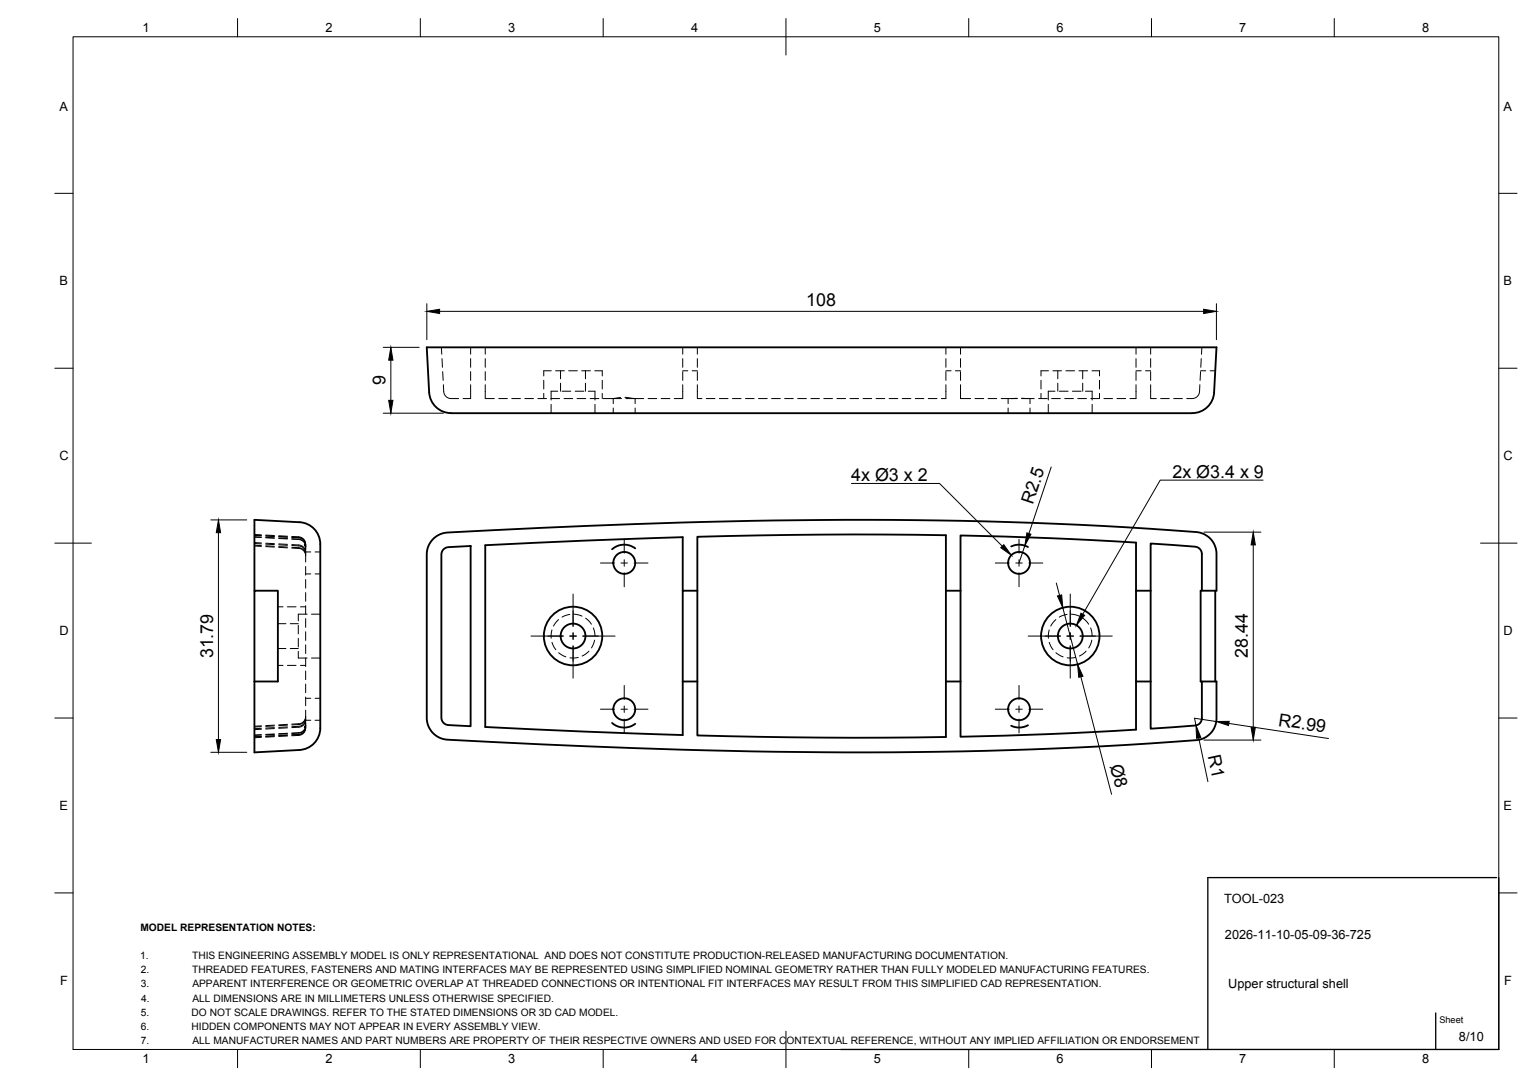
ISO-10303-21;
HEADER;
/* Generated by software containing ST-Developer
 * from STEP Tools, Inc. (www.steptools.com) 
 */

FILE_DESCRIPTION(
/* description */ (''),
/* implementation_level */ '2;1');

FILE_NAME(
/* name */ 'Upper structural shell.step',
/* time_stamp */ '2026-11-10T05:40:20-08:00',
/* author */ (''),
/* organization */ (''),
/* preprocessor_version */ 'ST-DEVELOPER v20.2',
/* originating_system */ 'Autodesk Translation Framework v15.17.0.0',
/* authorisation */ '');

FILE_SCHEMA (('AUTOMOTIVE_DESIGN { 1 0 10303 214 3 1 1 }'));
ENDSEC;

DATA;
#10=MECHANICAL_DESIGN_GEOMETRIC_PRESENTATION_REPRESENTATION('',(#575),#18580);
#76=SPHERICAL_SURFACE('',#6795,0.1);
#77=SPHERICAL_SURFACE('',#6798,0.0999999999999998);
#78=SPHERICAL_SURFACE('',#6802,0.0999999999999993);
#79=SPHERICAL_SURFACE('',#6806,0.1);
#80=SPHERICAL_SURFACE('',#6811,0.3);
#81=SPHERICAL_SURFACE('',#6815,0.3);
#82=SPHERICAL_SURFACE('',#6819,0.299999999999999);
#83=SPHERICAL_SURFACE('',#6824,0.3);
#92=B_SPLINE_SURFACE_WITH_KNOTS('',3,3,((#8816,#8817,#8818,#8819),(#8820,
#8821,#8822,#8823),(#8824,#8825,#8826,#8827),(#8828,#8829,#8830,#8831),
(#8832,#8833,#8834,#8835)),.UNSPECIFIED.,.F.,.F.,.F.,(4,1,4),(4,4),(0.,
0.571428571428571,1.),(1.0454440030657,3.44967454744645),.UNSPECIFIED.);
#93=B_SPLINE_SURFACE_WITH_KNOTS('',3,3,((#8908,#8909,#8910,#8911),(#8912,
#8913,#8914,#8915),(#8916,#8917,#8918,#8919),(#8920,#8921,#8922,#8923),
(#8924,#8925,#8926,#8927)),.UNSPECIFIED.,.F.,.F.,.F.,(4,1,4),(4,4),(0.,
0.571428571428571,1.),(7.24519303641511,9.95046872158573),.UNSPECIFIED.);
#94=B_SPLINE_SURFACE_WITH_KNOTS('',3,3,((#9789,#9790,#9791,#9792),(#9793,
#9794,#9795,#9796),(#9797,#9798,#9799,#9800),(#9801,#9802,#9803,#9804)),
 .UNSPECIFIED.,.F.,.F.,.F.,(4,4),(4,4),(0.0705535719740953,0.323522444336189),
(0.0117434863834119,0.684857763552191),.UNSPECIFIED.);
#95=B_SPLINE_SURFACE_WITH_KNOTS('',3,3,((#9809,#9810,#9811,#9812),(#9813,
#9814,#9815,#9816),(#9817,#9818,#9819,#9820),(#9821,#9822,#9823,#9824)),
 .UNSPECIFIED.,.F.,.F.,.F.,(4,4),(4,4),(0.0262419052680539,0.0545428296147404),
(0.0121538053864343,0.684980602226481),.UNSPECIFIED.);
#96=B_SPLINE_SURFACE_WITH_KNOTS('',3,3,((#9834,#9835,#9836,#9837),(#9838,
#9839,#9840,#9841),(#9842,#9843,#9844,#9845),(#9846,#9847,#9848,#9849),
(#9850,#9851,#9852,#9853)),.UNSPECIFIED.,.F.,.F.,.F.,(4,1,4),(4,4),(0.,
0.571428571428571,1.),(0.752061768057538,3.45733745322815),
 .UNSPECIFIED.);
#97=B_SPLINE_SURFACE_WITH_KNOTS('',3,3,((#9854,#9855,#9856,#9857),(#9858,
#9859,#9860,#9861),(#9862,#9863,#9864,#9865),(#9866,#9867,#9868,#9869),
(#9870,#9871,#9872,#9873)),.UNSPECIFIED.,.F.,.F.,.F.,(4,1,4),(4,4),(0.,
0.571428571428571,1.),(0.283259008618247,0.557056952888827),
 .UNSPECIFIED.);
#98=B_SPLINE_SURFACE_WITH_KNOTS('',3,3,((#9887,#9888,#9889,#9890),(#9891,
#9892,#9893,#9894),(#9895,#9896,#9897,#9898),(#9899,#9900,#9901,#9902)),
 .UNSPECIFIED.,.F.,.F.,.F.,(4,4),(4,4),(0.67647755566375,0.929446428026011),
(0.0117434863436937,0.684857763580381),.UNSPECIFIED.);
#99=B_SPLINE_SURFACE_WITH_KNOTS('',3,3,((#9903,#9904,#9905,#9906),(#9907,
#9908,#9909,#9910),(#9911,#9912,#9913,#9914),(#9915,#9916,#9917,#9918)),
 .UNSPECIFIED.,.F.,.F.,.F.,(4,4),(4,4),(0.945457170385156,0.973758094731946),
(0.0121538053598088,0.684980602226481),.UNSPECIFIED.);
#100=B_SPLINE_SURFACE_WITH_KNOTS('',3,3,((#10002,#10003,#10004,#10005),
(#10006,#10007,#10008,#10009),(#10010,#10011,#10012,#10013),(#10014,#10015,
#10016,#10017)),.UNSPECIFIED.,.F.,.F.,.F.,(4,4),(4,4),(0.341142793678372,
0.658675488550287),(0.0116221239297273,0.684255166525269),.UNSPECIFIED.);
#101=B_SPLINE_SURFACE_WITH_KNOTS('',3,3,((#10022,#10023,#10024,#10025),
(#10026,#10027,#10028,#10029),(#10030,#10031,#10032,#10033),(#10034,#10035,
#10036,#10037),(#10038,#10039,#10040,#10041)),.UNSPECIFIED.,.F.,.F.,.F.,
(4,1,4),(4,4),(0.,0.571428571428571,1.),(3.65450559744172,7.0548588409572),
 .UNSPECIFIED.);
#102=B_SPLINE_SURFACE_WITH_KNOTS('',3,3,((#10051,#10052,#10053,#10054),
(#10055,#10056,#10057,#10058),(#10059,#10060,#10061,#10062),(#10063,#10064,
#10065,#10066),(#10067,#10068,#10069,#10070)),.UNSPECIFIED.,.F.,.F.,.F.,
(4,1,4),(4,4),(0.,0.571428571428571,1.),(3.64767164868607,7.04802489220155),
 .UNSPECIFIED.);
#103=B_SPLINE_SURFACE_WITH_KNOTS('',3,3,((#10075,#10076,#10077,#10078),
(#10079,#10080,#10081,#10082),(#10083,#10084,#10085,#10086),(#10087,#10088,
#10089,#10090)),.UNSPECIFIED.,.F.,.F.,.F.,(4,4),(4,4),(0.341324511449716,
0.658857206321627),(0.0116221214776208,0.684255166525269),.UNSPECIFIED.);
#104=B_SPLINE_SURFACE_WITH_KNOTS('',3,3,((#10135,#10136,#10137,#10138),
(#10139,#10140,#10141,#10142),(#10143,#10144,#10145,#10146),(#10147,#10148,
#10149,#10150)),.UNSPECIFIED.,.F.,.F.,.F.,(4,4),(4,4),(0.676316266718331,
0.901708040522105),(0.0117102006467275,0.68495201331719),.UNSPECIFIED.);
#105=B_SPLINE_SURFACE_WITH_KNOTS('',3,3,((#10155,#10156,#10157,#10158),
(#10159,#10160,#10161,#10162),(#10163,#10164,#10165,#10166),(#10167,#10168,
#10169,#10170),(#10171,#10172,#10173,#10174)),.UNSPECIFIED.,.F.,.F.,.F.,
(4,1,4),(4,4),(0.,0.571428571428571,1.),(7.25285594219682,9.65708648657758),
 .UNSPECIFIED.);
#106=B_SPLINE_SURFACE_WITH_KNOTS('',3,3,((#10184,#10185,#10186,#10187),
(#10188,#10189,#10190,#10191),(#10192,#10193,#10194,#10195),(#10196,#10197,
#10198,#10199)),.UNSPECIFIED.,.F.,.F.,.F.,(4,4),(4,4),(0.0982919594778951,
0.323683733281714),(0.0117102006467272,0.68495201331719),.UNSPECIFIED.);
#107=B_SPLINE_SURFACE_WITH_KNOTS('',3,3,((#10274,#10275,#10276,#10277),
(#10278,#10279,#10280,#10281),(#10282,#10283,#10284,#10285),(#10286,#10287,
#10288,#10289)),.UNSPECIFIED.,.F.,.F.,.F.,(4,4),(4,4),(0.917922863855343,
0.974411608827007),(0.0122403473423911,0.685344304754238),.UNSPECIFIED.);
#108=B_SPLINE_SURFACE_WITH_KNOTS('',3,3,((#10299,#10300,#10301,#10302),
(#10303,#10304,#10305,#10306),(#10307,#10308,#10309,#10310),(#10311,#10312,
#10313,#10314),(#10315,#10316,#10317,#10318)),.UNSPECIFIED.,.F.,.F.,.F.,
(4,1,4),(4,4),(0.,0.571428571428571,1.),(9.85085636625011,10.4271318523291),
 .UNSPECIFIED.);
#109=B_SPLINE_SURFACE_WITH_KNOTS('',3,3,((#10332,#10333,#10334,#10335),
(#10336,#10337,#10338,#10339),(#10340,#10341,#10342,#10343),(#10344,#10345,
#10346,#10347)),.UNSPECIFIED.,.F.,.F.,.F.,(4,4),(4,4),(0.025588391172993,
0.0820771361446569),(0.0122403473423911,0.685344304754238),
 .UNSPECIFIED.);
#110=B_SPLINE_SURFACE_WITH_KNOTS('',3,3,((#10357,#10358,#10359,#10360),
(#10361,#10362,#10363,#10364),(#10365,#10366,#10367,#10368),(#10369,#10370,
#10371,#10372),(#10373,#10374,#10375,#10376)),.UNSPECIFIED.,.F.,.F.,.F.,
(4,1,4),(4,4),(0.,0.571428571428571,1.),(0.27539863731415,0.851674123393175),
 .UNSPECIFIED.);
#111=B_SPLINE_SURFACE_WITH_KNOTS('',3,3,((#10390,#10391,#10392,#10393),
(#10394,#10395,#10396,#10397),(#10398,#10399,#10400,#10401),(#10402,#10403,
#10404,#10405),(#10406,#10407,#10408,#10409)),.UNSPECIFIED.,.F.,.F.,.F.,
(4,1,4),(4,4),(0.,0.571428571428571,1.),(0.00944995813270487,0.618489359031386),
 .UNSPECIFIED.);
#112=B_SPLINE_SURFACE_WITH_KNOTS('',3,3,((#10416,#10417,#10418,#10419),
(#10420,#10421,#10422,#10423),(#10424,#10425,#10426,#10427),(#10428,#10429,
#10430,#10431),(#10432,#10433,#10434,#10435)),.UNSPECIFIED.,.F.,.F.,.F.,
(4,1,4),(4,4),(0.,0.571428571428571,1.),(0.00908570715245136,0.618164468641375),
 .UNSPECIFIED.);
#113=B_SPLINE_SURFACE_WITH_KNOTS('',3,3,((#10440,#10441,#10442,#10443),
(#10444,#10445,#10446,#10447),(#10448,#10449,#10450,#10451),(#10452,#10453,
#10454,#10455),(#10456,#10457,#10458,#10459)),.UNSPECIFIED.,.F.,.F.,.F.,
(4,1,4),(4,4),(0.,0.571428571428571,1.),(0.0091183540525243,0.618164468641375),
 .UNSPECIFIED.);
#114=B_SPLINE_SURFACE_WITH_KNOTS('',3,3,((#10464,#10465,#10466,#10467),
(#10468,#10469,#10470,#10471),(#10472,#10473,#10474,#10475),(#10476,#10477,
#10478,#10479),(#10480,#10481,#10482,#10483)),.UNSPECIFIED.,.F.,.F.,.F.,
(4,1,4),(4,4),(0.,0.571428571428571,1.),(10.1454735367545,10.419271481025),
 .UNSPECIFIED.);
#115=B_SPLINE_SURFACE_WITH_KNOTS('',3,3,((#10484,#10485,#10486,#10487),
(#10488,#10489,#10490,#10491),(#10492,#10493,#10494,#10495),(#10496,#10497,
#10498,#10499),(#10500,#10501,#10502,#10503)),.UNSPECIFIED.,.F.,.F.,.F.,
(4,1,4),(4,4),(0.,0.571428571428571,1.),(0.0094045468285345,0.618489359031386),
 .UNSPECIFIED.);
#116=B_SPLINE_SURFACE_WITH_KNOTS('',3,3,((#10529,#10530,#10531,#10532),
(#10533,#10534,#10535,#10536),(#10537,#10538,#10539,#10540),(#10541,#10542,
#10543,#10544),(#10545,#10546,#10547,#10548)),.UNSPECIFIED.,.F.,.F.,.F.,
(4,1,4),(4,4),(0.,0.571428571428571,1.),(-0.00535061636073277,0.618489359031386),
 .UNSPECIFIED.);
#117=B_SPLINE_SURFACE_WITH_KNOTS('',3,3,((#10567,#10568,#10569,#10570,#10571),
(#10572,#10573,#10574,#10575,#10576),(#10577,#10578,#10579,#10580,#10581),
(#10582,#10583,#10584,#10585,#10586),(#10587,#10588,#10589,#10590,#10591)),
 .UNSPECIFIED.,.F.,.F.,.F.,(4,1,4),(4,1,4),(0.,0.571428571428571,1.),(0.283259008618247,
4.63063308449434,10.4271318523291),.UNSPECIFIED.);
#118=B_SPLINE_SURFACE_WITH_KNOTS('',3,3,((#10602,#10603,#10604,#10605),
(#10606,#10607,#10608,#10609),(#10610,#10611,#10612,#10613),(#10614,#10615,
#10616,#10617),(#10618,#10619,#10620,#10621)),.UNSPECIFIED.,.F.,.F.,.F.,
(4,1,4),(4,4),(0.,0.571428571428571,1.),(-0.00578978989683084,0.618164468641375),
 .UNSPECIFIED.);
#119=B_SPLINE_SURFACE_WITH_KNOTS('',3,3,((#10630,#10631,#10632,#10633),
(#10634,#10635,#10636,#10637),(#10638,#10639,#10640,#10641),(#10642,#10643,
#10644,#10645),(#10646,#10647,#10648,#10649)),.UNSPECIFIED.,.F.,.F.,.F.,
(4,1,4),(4,4),(0.,0.571428571428571,1.),(-0.00569189159989896,0.618164468641375),
 .UNSPECIFIED.);
#120=B_SPLINE_SURFACE_WITH_KNOTS('',3,3,((#10658,#10659,#10660,#10661,#10662),
(#10663,#10664,#10665,#10666,#10667),(#10668,#10669,#10670,#10671,#10672),
(#10673,#10674,#10675,#10676,#10677),(#10678,#10679,#10680,#10681,#10682)),
 .UNSPECIFIED.,.F.,.F.,.F.,(4,1,4),(4,1,4),(0.,0.571428571428571,1.),(0.27539863731415,
4.62277271319024,10.419271481025),.UNSPECIFIED.);
#121=B_SPLINE_SURFACE_WITH_KNOTS('',3,3,((#10693,#10694,#10695,#10696),
(#10697,#10698,#10699,#10700),(#10701,#10702,#10703,#10704),(#10705,#10706,
#10707,#10708),(#10709,#10710,#10711,#10712)),.UNSPECIFIED.,.F.,.F.,.F.,
(4,1,4),(4,4),(0.,0.571428571428571,1.),(-0.0054868135546625,0.618489359031386),
 .UNSPECIFIED.);
#122=B_SPLINE_SURFACE_WITH_KNOTS('',3,3,((#10721,#10722,#10723,#10724),
(#10725,#10726,#10727,#10728),(#10729,#10730,#10731,#10732),(#10733,#10734,
#10735,#10736)),.UNSPECIFIED.,.F.,.F.,.F.,(4,4),(4,4),(0.026239262514127,
0.974414173651419),(0.,0.685344304754238),.UNSPECIFIED.);
#123=B_SPLINE_SURFACE_WITH_KNOTS('',3,3,((#10739,#10740,#10741,#10742),
(#10743,#10744,#10745,#10746),(#10747,#10748,#10749,#10750),(#10751,#10752,
#10753,#10754)),.UNSPECIFIED.,.F.,.F.,.F.,(4,4),(4,4),(0.0255858263485814,
0.973760737485873),(0.,0.685344304754238),.UNSPECIFIED.);
#172=B_SPLINE_CURVE_WITH_KNOTS('',3,(#8715,#8716,#8717,#8718,#8719,#8720,
#8721,#8722,#8723,#8724,#8725,#8726,#8727,#8728,#8729,#8730,#8731,#8732,
#8733,#8734,#8735,#8736,#8737,#8738),.UNSPECIFIED.,.F.,.F.,(4,2,2,2,2,2,
2,2,2,2,2,4),(-0.337265338267783,-0.250544943628509,-0.208272806508042,
-0.186542211788094,-0.176382978682897,-0.170925844043069,-0.16639450677335,
-0.161077381235501,-0.15182241135393,-0.115009181549223,-0.030206004227969,
0.),.UNSPECIFIED.);
#173=B_SPLINE_CURVE_WITH_KNOTS('',3,(#8743,#8744,#8745,#8746,#8747,#8748,
#8749,#8750,#8751,#8752,#8753,#8754,#8755,#8756,#8757,#8758,#8759,#8760,
#8761,#8762),.UNSPECIFIED.,.F.,.F.,(4,2,2,2,2,2,2,2,2,4),(-0.240982594686416,
-0.16829976149504,-0.141836598208813,-0.129116059226128,-0.121962912034391,
-0.115857591426886,-0.108506552485159,-0.0948769875819265,-0.0364654790774683,
0.),.UNSPECIFIED.);
#174=B_SPLINE_CURVE_WITH_KNOTS('',3,(#8767,#8768,#8769,#8770,#8771,#8772,
#8773,#8774,#8775,#8776,#8777,#8778,#8779,#8780,#8781,#8782,#8783,#8784,
#8785,#8786),.UNSPECIFIED.,.F.,.F.,(4,2,2,2,2,2,2,2,2,4),(-0.240981214998207,
-0.168303541671295,-0.141841407502325,-0.129121097580905,-0.121968013294536,
-0.115862708924237,-0.108511643765797,-0.0948818976588229,-0.0364681276985956,
0.),.UNSPECIFIED.);
#175=B_SPLINE_CURVE_WITH_KNOTS('',3,(#8791,#8792,#8793,#8794,#8795,#8796,
#8797,#8798,#8799,#8800,#8801,#8802,#8803,#8804,#8805,#8806,#8807,#8808,
#8809,#8810,#8811,#8812,#8813,#8814),.UNSPECIFIED.,.F.,.F.,(4,2,2,2,2,2,
2,2,2,2,2,4),(-0.337269388373684,-0.250545316912909,-0.208282401844766,
-0.186554569827561,-0.176396213396297,-0.17093921790305,-0.16640782243471,
-0.161090427650893,-0.151834477986603,-0.115010808423941,-0.0302102096065556,
0.),.UNSPECIFIED.);
#176=B_SPLINE_CURVE_WITH_KNOTS('',3,(#8837,#8838,#8839,#8840),
 .UNSPECIFIED.,.F.,.F.,(4,4),(1.0454440030657,2.52465537163019),
 .UNSPECIFIED.);
#177=B_SPLINE_CURVE_WITH_KNOTS('',3,(#8842,#8843,#8844,#8845,#8846,#8847,
#8848,#8849,#8850,#8851,#8852,#8853,#8854,#8855,#8856,#8857,#8858,#8859,
#8860,#8861,#8862,#8863,#8864,#8865,#8866,#8867,#8868,#8869),
 .UNSPECIFIED.,.F.,.F.,(4,3,3,3,3,3,3,3,3,4),(-0.152193408756968,-0.128427023368412,
-0.115107736263918,-0.0911810900745799,-0.0780377802127556,-0.0652031397886901,
-0.0414031558437525,-0.0389949527774582,-0.0152076153333754,0.),
 .UNSPECIFIED.);
#178=B_SPLINE_CURVE_WITH_KNOTS('',3,(#8871,#8872,#8873,#8874),
 .UNSPECIFIED.,.F.,.F.,(4,4),(-3.44967454744645,-1.05170160817356),
 .UNSPECIFIED.);
#179=B_SPLINE_CURVE_WITH_KNOTS('',3,(#8876,#8877,#8878,#8879,#8880,#8881,
#8882,#8883,#8884,#8885,#8886,#8887,#8888,#8889,#8890,#8891,#8892,#8893,
#8894,#8895,#8896,#8897,#8898,#8899,#8900,#8901,#8902,#8903),
 .UNSPECIFIED.,.F.,.F.,(4,3,3,3,3,3,3,3,3,4),(-0.152278960443096,-0.128503570101575,
-0.115218572146868,-0.09145408274965,-0.0870214650669139,-0.0781562978024333,
-0.0542566895399357,-0.03908030849237,-0.0153296112319379,0.),
 .UNSPECIFIED.);
#180=B_SPLINE_CURVE_WITH_KNOTS('',3,(#8904,#8905,#8906,#8907),
 .UNSPECIFIED.,.F.,.F.,(4,4),(2.75501813708031,3.4476340663212),
 .UNSPECIFIED.);
#181=B_SPLINE_CURVE_WITH_KNOTS('',3,(#8929,#8930,#8931,#8932),
 .UNSPECIFIED.,.F.,.F.,(4,4),(7.24810383506675,7.89761558728778),
 .UNSPECIFIED.);
#182=B_SPLINE_CURVE_WITH_KNOTS('',3,(#8934,#8935,#8936,#8937,#8938,#8939,
#8940,#8941,#8942,#8943,#8944,#8945,#8946,#8947,#8948,#8949,#8950,#8951,
#8952,#8953,#8954,#8955,#8956,#8957,#8958,#8959,#8960,#8961),
 .UNSPECIFIED.,.F.,.F.,(4,3,3,3,3,3,3,3,3,4),(-0.152278869104567,-0.128548794904564,
-0.115192257893812,-0.0912773536606376,-0.0781090575823055,-0.0652724057916263,
-0.0414819581560496,-0.0390493575290778,-0.015259721743698,0.),
 .UNSPECIFIED.);
#183=B_SPLINE_CURVE_WITH_KNOTS('',3,(#8963,#8964,#8965,#8966),
 .UNSPECIFIED.,.F.,.F.,(4,4),(-9.94532343034734,-7.24519303641511),
 .UNSPECIFIED.);
#184=B_SPLINE_CURVE_WITH_KNOTS('',3,(#8968,#8969,#8970,#8971,#8972,#8973,
#8974,#8975,#8976,#8977,#8978,#8979,#8980,#8981,#8982,#8983,#8984,#8985,
#8986,#8987,#8988,#8989,#8990,#8991,#8992,#8993,#8994,#8995),
 .UNSPECIFIED.,.F.,.F.,(4,3,3,3,3,3,3,3,3,4),(-0.152181623618259,-0.128410404494075,
-0.115248188224843,-0.0914746846046984,-0.0869904866333268,-0.0783028696190655,
-0.0543945376065823,-0.0391651209697638,-0.0153884182770307,0.),
 .UNSPECIFIED.);
#185=B_SPLINE_CURVE_WITH_KNOTS('',3,(#8996,#8997,#8998,#8999),
 .UNSPECIFIED.,.F.,.F.,(4,4),(8.21380824320284,9.95046871680089),
 .UNSPECIFIED.);
#186=B_SPLINE_CURVE_WITH_KNOTS('',3,(#9002,#9003,#9004,#9005),
 .UNSPECIFIED.,.F.,.F.,(4,4),(2.80491490332713,3.45442665446657),
 .UNSPECIFIED.);
#187=B_SPLINE_CURVE_WITH_KNOTS('',3,(#9009,#9010,#9011,#9012),
 .UNSPECIFIED.,.F.,.F.,(4,4),(0.752061768057538,2.48872224644044),
 .UNSPECIFIED.);
#188=B_SPLINE_CURVE_WITH_KNOTS('',3,(#9160,#9161,#9162,#9163,#9164,#9165),
 .UNSPECIFIED.,.F.,.F.,(4,2,4),(-0.606700505977711,-0.303383635264422,-0.000339350725729326),
 .UNSPECIFIED.);
#189=B_SPLINE_CURVE_WITH_KNOTS('',3,(#9166,#9167,#9168,#9169,#9170,#9171,
#9172,#9173,#9174,#9175,#9176,#9177,#9178,#9179,#9180,#9181,#9182,#9183,
#9184,#9185,#9186,#9187,#9188,#9189,#9190,#9191,#9192,#9193),
 .UNSPECIFIED.,.F.,.F.,(4,3,3,3,3,3,3,3,3,4),(-0.152173579228948,-0.128423230539522,
-0.115115104157663,-0.0911927259648815,-0.0780672068328041,-0.0652082609452843,
-0.0414117413801899,-0.0390174000215468,-0.0152300060615686,0.),
 .UNSPECIFIED.);
#190=B_SPLINE_CURVE_WITH_KNOTS('',3,(#9194,#9195,#9196,#9197,#9198,#9199),
 .UNSPECIFIED.,.F.,.F.,(4,2,4),(-0.606471894652381,-0.303383500305553,-0.00011071898471493),
 .UNSPECIFIED.);
#191=B_SPLINE_CURVE_WITH_KNOTS('',3,(#9203,#9204,#9205,#9206,#9207,#9208),
 .UNSPECIFIED.,.F.,.F.,(4,2,4),(-0.606240625011114,-0.303433113375332,-0.00010938105916114),
 .UNSPECIFIED.);
#192=B_SPLINE_CURVE_WITH_KNOTS('',3,(#9210,#9211,#9212,#9213,#9214,#9215,
#9216,#9217,#9218,#9219,#9220,#9221,#9222,#9223,#9224,#9225,#9226,#9227,
#9228,#9229,#9230,#9231,#9232,#9233,#9234,#9235,#9236,#9237),
 .UNSPECIFIED.,.F.,.F.,(4,3,3,3,3,3,3,3,3,4),(-0.152281454644235,-0.128508102092242,
-0.115234945630277,-0.0914677943501604,-0.0870276017853555,-0.0781846052914712,
-0.0542821334115454,-0.0390966859411886,-0.0153419673568312,0.),
 .UNSPECIFIED.);
#193=B_SPLINE_CURVE_WITH_KNOTS('',3,(#9239,#9240,#9241,#9242,#9243,#9244),
 .UNSPECIFIED.,.F.,.F.,(4,2,4),(-0.606758573154242,-0.303433157101101,-0.000627306481538803),
 .UNSPECIFIED.);
#194=B_SPLINE_CURVE_WITH_KNOTS('',3,(#9250,#9251,#9252,#9253,#9254,#9255),
 .UNSPECIFIED.,.F.,.F.,(4,2,4),(-0.60617382748,-0.303436117212405,-7.2700296824213E-5),
 .UNSPECIFIED.);
#195=B_SPLINE_CURVE_WITH_KNOTS('',3,(#9257,#9258,#9259,#9260,#9261,#9262,
#9263,#9264,#9265,#9266,#9267,#9268,#9269,#9270,#9271,#9272,#9273,#9274,
#9275,#9276,#9277,#9278,#9279,#9280,#9281,#9282,#9283,#9284),
 .UNSPECIFIED.,.F.,.F.,(4,3,3,3,3,3,3,3,3,4),(-0.152282154327755,-0.128558036203745,
-0.115201429639692,-0.0912891813973639,-0.0781219052297615,-0.065279687589213,
-0.0414913146723999,-0.0390591331507366,-0.0152683745546824,0.),
 .UNSPECIFIED.);
#196=B_SPLINE_CURVE_WITH_KNOTS('',3,(#9288,#9289,#9290,#9291,#9292,#9293,
#9294,#9295,#9296,#9297,#9298,#9299,#9300,#9301,#9302,#9303,#9304,#9305,
#9306,#9307,#9308,#9309,#9310,#9311,#9312,#9313,#9314,#9315),
 .UNSPECIFIED.,.F.,.F.,(4,3,3,3,3,3,3,3,3,4),(-0.152283066055976,-0.128508717930245,
-0.115216472798554,-0.091451700383826,-0.087022506454752,-0.0781485278686168,
-0.0542483994686567,-0.0390758108455304,-0.0153274175274101,0.),
 .UNSPECIFIED.);
#197=B_SPLINE_CURVE_WITH_KNOTS('',3,(#9317,#9318,#9319,#9320,#9321,#9322),
 .UNSPECIFIED.,.F.,.F.,(4,2,4),(-0.606800264911061,-0.303436147592132,-0.000699137727853738),
 .UNSPECIFIED.);
#198=B_SPLINE_CURVE_WITH_KNOTS('',3,(#9327,#9328,#9329,#9330,#9331,#9332),
 .UNSPECIFIED.,.F.,.F.,(4,2,4),(-0.606915279655722,-0.30363236403835,-0.000516487074480598),
 .UNSPECIFIED.);
#199=B_SPLINE_CURVE_WITH_KNOTS('',3,(#9336,#9337,#9338,#9339,#9340,#9341,
#9342,#9343,#9344,#9345,#9346,#9347,#9348,#9349,#9350,#9351,#9352,#9353,
#9354,#9355,#9356,#9357,#9358,#9359,#9360,#9361,#9362,#9363),
 .UNSPECIFIED.,.F.,.F.,(4,3,3,3,3,3,3,3,3,4),(-0.152205325335401,-0.128433618138404,
-0.115304790388008,-0.091527299141506,-0.0870178586418932,-0.0783866443643876,
-0.0544751548276533,-0.0392137310602028,-0.0154203878854647,0.),
 .UNSPECIFIED.);
#200=B_SPLINE_CURVE_WITH_KNOTS('',3,(#9365,#9366,#9367,#9368,#9369,#9370),
 .UNSPECIFIED.,.F.,.F.,(4,2,4),(-0.606752424187958,-0.303632696349781,-0.000353591088346872),
 .UNSPECIFIED.);
#201=B_SPLINE_CURVE_WITH_KNOTS('',3,(#9376,#9377,#9378,#9379),
 .UNSPECIFIED.,.F.,.F.,(4,4),(0.0116023361771303,0.618489359031386),
 .UNSPECIFIED.);
#202=B_SPLINE_CURVE_WITH_KNOTS('',3,(#9383,#9384,#9385,#9386),
 .UNSPECIFIED.,.F.,.F.,(4,4),(-0.618489359031386,-0.01160233617713),
 .UNSPECIFIED.);
#203=B_SPLINE_CURVE_WITH_KNOTS('',3,(#9389,#9390,#9391,#9392),
 .UNSPECIFIED.,.F.,.F.,(4,4),(7.01593971618694,9.71770560667459),
 .UNSPECIFIED.);
#204=B_SPLINE_CURVE_WITH_KNOTS('',3,(#9393,#9394,#9395,#9396),
 .UNSPECIFIED.,.F.,.F.,(4,4),(0.505945342046796,3.20718651982575),
 .UNSPECIFIED.);
#205=B_SPLINE_CURVE_WITH_KNOTS('',3,(#9399,#9400,#9401,#9402,#9403,#9404,
#9405),.UNSPECIFIED.,.F.,.F.,(4,3,4),(3.40717417387402,5.11170895874517,
6.80746068626633),.UNSPECIFIED.);
#206=B_SPLINE_CURVE_WITH_KNOTS('',3,(#9408,#9409,#9410,#9411),
 .UNSPECIFIED.,.F.,.F.,(4,4),(7.00766573366377,9.41198845520559),
 .UNSPECIFIED.);
#207=B_SPLINE_CURVE_WITH_KNOTS('',3,(#9415,#9416,#9417,#9418),
 .UNSPECIFIED.,.F.,.F.,(4,4),(9.61248784142317,10.2217363065808),
 .UNSPECIFIED.);
#208=B_SPLINE_CURVE_WITH_KNOTS('',3,(#9419,#9420,#9421,#9422,#9423,#9424,
#9425,#9426,#9427,#9428,#9429,#9430,#9431,#9432,#9433,#9434,#9435,#9436,
#9437,#9438,#9439,#9440,#9441,#9442,#9443,#9444,#9445,#9446),
 .UNSPECIFIED.,.F.,.F.,(4,3,3,3,3,3,3,3,3,4),(0.,0.0238103109064959,0.0390781362249314,
0.0628635086275546,0.0641230352384255,0.0780643700703951,0.101962174814111,
0.113803522271848,0.137549611554782,0.149564734365165),.UNSPECIFIED.);
#209=B_SPLINE_CURVE_WITH_KNOTS('',3,(#9450,#9451,#9452,#9453,#9454,#9455,
#9456,#9457,#9458,#9459,#9460,#9461,#9462,#9463,#9464,#9465,#9466,#9467,
#9468,#9469,#9470,#9471,#9472,#9473,#9474,#9475,#9476,#9477,#9478,#9479,
#9480),.UNSPECIFIED.,.F.,.F.,(4,3,3,3,3,3,3,3,3,3,4),(0.,0.0535521515156599,
0.107729685495911,0.117233338918226,0.171447998942947,0.1923696899792,0.234191611538245,
0.288659693466396,0.341410301570312,0.395549383747909,0.448696573746633),
 .UNSPECIFIED.);
#210=B_SPLINE_CURVE_WITH_KNOTS('',3,(#9482,#9483,#9484,#9485),
 .UNSPECIFIED.,.F.,.F.,(4,4),(0.0255858263485814,0.973760737485873),
 .UNSPECIFIED.);
#211=B_SPLINE_CURVE_WITH_KNOTS('',3,(#9487,#9488,#9489,#9490,#9491,#9492,
#9493,#9494,#9495,#9496,#9497,#9498,#9499,#9500,#9501,#9502,#9503,#9504,
#9505,#9506,#9507,#9508,#9509,#9510,#9511,#9512,#9513,#9514,#9515,#9516,
#9517),.UNSPECIFIED.,.F.,.F.,(4,3,3,3,3,3,3,3,3,3,4),(0.,0.0535144560117858,
0.107726856902975,0.117300577410231,0.171517675930231,0.195438847090422,
0.234297456941738,0.289665153342662,0.345032849743585,0.40043206955427,
0.455831289364955),.UNSPECIFIED.);
#212=B_SPLINE_CURVE_WITH_KNOTS('',3,(#9521,#9522,#9523,#9524,#9525,#9526,
#9527,#9528,#9529,#9530,#9531,#9532,#9533,#9534,#9535,#9536,#9537,#9538,
#9539,#9540,#9541,#9542,#9543,#9544,#9545,#9546,#9547,#9548,#9549,#9550,
#9551),.UNSPECIFIED.,.F.,.F.,(4,3,3,3,3,3,3,3,3,3,4),(0.,0.053505543180391,
0.107714168832353,0.117253997025819,0.171473395203321,0.195418854185489,
0.234223199196375,0.289607016015183,0.344990832833991,0.400409777473312,
0.455828722112633),.UNSPECIFIED.);
#213=B_SPLINE_CURVE_WITH_KNOTS('',3,(#9553,#9554,#9555,#9556),
 .UNSPECIFIED.,.F.,.F.,(4,4),(0.0262392625141271,0.974414173651419),
 .UNSPECIFIED.);
#214=B_SPLINE_CURVE_WITH_KNOTS('',3,(#9558,#9559,#9560,#9561,#9562,#9563,
#9564,#9565,#9566,#9567,#9568,#9569,#9570,#9571,#9572,#9573,#9574,#9575,
#9576,#9577,#9578,#9579,#9580,#9581,#9582,#9583,#9584,#9585,#9586,#9587,
#9588),.UNSPECIFIED.,.F.,.F.,(4,3,3,3,3,3,3,3,3,3,4),(0.,0.0535648734523888,
0.107747221190676,0.117299947751206,0.171510987106922,0.192397607227928,
0.234296687348373,0.288768001369001,0.341469499352622,0.395597672314973,
0.448700135162036),.UNSPECIFIED.);
#215=B_SPLINE_CURVE_WITH_KNOTS('',3,(#9591,#9592,#9593,#9594,#9595,#9596,
#9597,#9598,#9599,#9600,#9601,#9602,#9603,#9604,#9605,#9606,#9607,#9608,
#9609,#9610,#9611,#9612,#9613,#9614,#9615),.UNSPECIFIED.,.F.,.F.,(4,3,3,
3,3,3,3,3,4),(0.,0.0238141989470671,0.0391004231578824,0.0641320992313133,
0.0780996136084711,0.101998806889826,0.113823260594808,0.137564745199532,
0.149565921982294),.UNSPECIFIED.);
#216=B_SPLINE_CURVE_WITH_KNOTS('',3,(#9617,#9618,#9619,#9620),
 .UNSPECIFIED.,.F.,.F.,(4,4),(2.76692059912875E-5,0.609394470571143),
 .UNSPECIFIED.);
#217=B_SPLINE_CURVE_WITH_KNOTS('',3,(#9623,#9624,#9625,#9626),
 .UNSPECIFIED.,.F.,.F.,(4,4),(0.809932799154201,3.21472245120952),
 .UNSPECIFIED.);
#218=B_SPLINE_CURVE_WITH_KNOTS('',3,(#9629,#9630,#9631,#9632,#9633,#9634,
#9635),.UNSPECIFIED.,.F.,.F.,(4,3,4),(3.41496637450242,5.11093193409745,
6.81591321610411),.UNSPECIFIED.);
#219=B_SPLINE_CURVE_WITH_KNOTS('',3,(#9639,#9640,#9641,#9642),
 .UNSPECIFIED.,.F.,.F.,(4,4),(9.91798263530139,10.2237206759544),
 .UNSPECIFIED.);
#220=B_SPLINE_CURVE_WITH_KNOTS('',3,(#9644,#9645,#9646,#9647,#9648,#9649,
#9650,#9651,#9652,#9653,#9654,#9655,#9656,#9657,#9658,#9659,#9660,#9661,
#9662,#9663,#9664,#9665,#9666,#9667,#9668,#9669,#9670,#9671),
 .UNSPECIFIED.,.F.,.F.,(4,3,3,3,3,3,3,3,3,4),(0.,0.023807020713713,0.039085080816122,
0.0628703378723092,0.0651394887354207,0.0780750047750988,0.101981498769656,
0.114997221725907,0.138748569029605,0.151942344104828),.UNSPECIFIED.);
#221=B_SPLINE_CURVE_WITH_KNOTS('',3,(#9675,#9676,#9677,#9678,#9679,#9680,
#9681,#9682,#9683,#9684,#9685,#9686,#9687,#9688,#9689,#9690,#9691,#9692,
#9693,#9694,#9695,#9696,#9697,#9698,#9699,#9700,#9701,#9702),
 .UNSPECIFIED.,.F.,.F.,(4,3,3,3,3,3,3,3,3,4),(0.,0.0238098191818892,0.0391006681981376,
0.0628849269680955,0.0651459659463291,0.0780999162396042,0.102007524384594,
0.115011225379555,0.138759376430353,0.151943200125079),.UNSPECIFIED.);
#222=B_SPLINE_CURVE_WITH_KNOTS('',3,(#9704,#9705,#9706,#9707),
 .UNSPECIFIED.,.F.,.F.,(4,4),(2.85486020485948E-5,0.305707210239178),
 .UNSPECIFIED.);
#223=B_SPLINE_CURVE_WITH_KNOTS('',3,(#9717,#9718,#9719,#9720,#9721,#9722),
 .UNSPECIFIED.,.F.,.F.,(4,2,4),(-0.606446248197249,-0.303383959626182,-6.4365448350312E-5),
 .UNSPECIFIED.);
#224=B_SPLINE_CURVE_WITH_KNOTS('',3,(#9724,#9725,#9726,#9727,#9728,#9729),
 .UNSPECIFIED.,.F.,.F.,(4,2,4),(-0.60675170080159,-0.303384112192838,-0.000369837888147484),
 .UNSPECIFIED.);
#225=B_SPLINE_CURVE_WITH_KNOTS('',3,(#9731,#9732,#9733,#9734,#9735,#9736,
#9737,#9738,#9739,#9740,#9741,#9742,#9743,#9744,#9745,#9746,#9747,#9748,
#9749,#9750,#9751,#9752,#9753,#9754,#9755,#9756,#9757,#9758),
 .UNSPECIFIED.,.F.,.F.,(4,3,3,3,3,3,3,3,3,4),(-0.152162866344201,-0.128411131698784,
-0.115108013904405,-0.0911850729173883,-0.0780642464630149,-0.0652023242402653,
-0.0414053499882389,-0.0390151293250392,-0.0152279490549848,0.),
 .UNSPECIFIED.);
#226=B_SPLINE_CURVE_WITH_KNOTS('',3,(#9761,#9762,#9763,#9764,#9765,#9766,
#9767,#9768,#9769,#9770,#9771,#9772,#9773,#9774,#9775,#9776,#9777,#9778,
#9779,#9780,#9781,#9782,#9783,#9784,#9785,#9786,#9787,#9788),
 .UNSPECIFIED.,.F.,.F.,(4,3,3,3,3,3,3,3,3,4),(-0.152171297476962,-0.128400300768352,
-0.115247520946962,-0.0914735511738372,-0.0869860114952295,-0.0783112904282795,
-0.0544025203706761,-0.0391699941254272,-0.015391764586027,0.),
 .UNSPECIFIED.);
#227=B_SPLINE_CURVE_WITH_KNOTS('',3,(#9805,#9806,#9807,#9808),
 .UNSPECIFIED.,.F.,.F.,(4,4),(-3.45733745322815,-0.757207059295936),
 .UNSPECIFIED.);
#228=B_SPLINE_CURVE_WITH_KNOTS('',3,(#9826,#9827,#9828,#9829),
 .UNSPECIFIED.,.F.,.F.,(4,4),(-0.557056952888827,-0.283259008618247),
 .UNSPECIFIED.);
#229=B_SPLINE_CURVE_WITH_KNOTS('',3,(#9830,#9831,#9832,#9833),
 .UNSPECIFIED.,.F.,.F.,(4,4),(-0.618164468641375,-0.0110156167597059),
 .UNSPECIFIED.);
#230=B_SPLINE_CURVE_WITH_KNOTS('',3,(#9875,#9876,#9877,#9878),
 .UNSPECIFIED.,.F.,.F.,(4,4),(0.283259011433088,0.551788488929761),
 .UNSPECIFIED.);
#231=B_SPLINE_CURVE_WITH_KNOTS('',3,(#9882,#9883,#9884,#9885),
 .UNSPECIFIED.,.F.,.F.,(4,4),(10.1507419987596,10.419271481025),
 .UNSPECIFIED.);
#232=B_SPLINE_CURVE_WITH_KNOTS('',3,(#9920,#9921,#9922,#9923),
 .UNSPECIFIED.,.F.,.F.,(4,4),(0.0110156167597055,0.618164468641375),
 .UNSPECIFIED.);
#233=B_SPLINE_CURVE_WITH_KNOTS('',3,(#9924,#9925,#9926,#9927),
 .UNSPECIFIED.,.F.,.F.,(4,4),(-10.419271481025,-10.1454735367545),
 .UNSPECIFIED.);
#234=B_SPLINE_CURVE_WITH_KNOTS('',3,(#9930,#9931,#9932,#9933,#9934,#9935),
 .UNSPECIFIED.,.F.,.F.,(4,2,4),(-0.606211482799139,-0.303431960476852,-9.19895310989571E-5),
 .UNSPECIFIED.);
#235=B_SPLINE_CURVE_WITH_KNOTS('',3,(#9937,#9938,#9939,#9940,#9941,#9942,
#9943,#9944,#9945,#9946,#9947,#9948,#9949,#9950,#9951,#9952,#9953,#9954,
#9955,#9956,#9957,#9958,#9959,#9960,#9961,#9962,#9963,#9964),
 .UNSPECIFIED.,.F.,.F.,(4,3,3,3,3,3,3,3,3,4),(-0.152283340966725,-0.128554242174982,
-0.115196092098682,-0.0912819860997417,-0.0781117853096875,-0.0652755629514801,
-0.0414857317972147,-0.039051434275634,-0.0152612146291672,0.),
 .UNSPECIFIED.);
#236=B_SPLINE_CURVE_WITH_KNOTS('',3,(#9968,#9969,#9970,#9971,#9972,#9973,
#9974,#9975,#9976,#9977,#9978,#9979,#9980,#9981,#9982,#9983,#9984,#9985,
#9986,#9987,#9988,#9989,#9990,#9991,#9992,#9993,#9994,#9995),
 .UNSPECIFIED.,.F.,.F.,(4,3,3,3,3,3,3,3,3,4),(-0.152285570909379,-0.128511627155755,
-0.115232904621082,-0.0914664612111958,-0.0870286654075453,-0.0781769338106538,
-0.0542752301960614,-0.039092246575741,-0.0153386136911565,0.),
 .UNSPECIFIED.);
#237=B_SPLINE_CURVE_WITH_KNOTS('',3,(#9996,#9997,#9998,#9999,#10000,#10001),
 .UNSPECIFIED.,.F.,.F.,(4,2,4),(-0.606773318344362,-0.303431998667662,-0.000653802131222458),
 .UNSPECIFIED.);
#238=B_SPLINE_CURVE_WITH_KNOTS('',3,(#10018,#10019,#10020,#10021),
 .UNSPECIFIED.,.F.,.F.,(4,4),(-7.05313168653828,-3.6572084986735),
 .UNSPECIFIED.);
#239=B_SPLINE_CURVE_WITH_KNOTS('',3,(#10042,#10043,#10044,#10045),
 .UNSPECIFIED.,.F.,.F.,(4,4),(3.65450559744172,7.0548588409572),
 .UNSPECIFIED.);
#240=B_SPLINE_CURVE_WITH_KNOTS('',3,(#10047,#10048,#10049,#10050),
 .UNSPECIFIED.,.F.,.F.,(4,4),(3.64767164868607,7.04802489220155),
 .UNSPECIFIED.);
#241=B_SPLINE_CURVE_WITH_KNOTS('',3,(#10071,#10072,#10073,#10074),
 .UNSPECIFIED.,.F.,.F.,(4,4),(-7.04532199096977,-3.64939880310499),
 .UNSPECIFIED.);
#242=B_SPLINE_CURVE_WITH_KNOTS('',3,(#10093,#10094,#10095,#10096,#10097,
#10098),.UNSPECIFIED.,.F.,.F.,(4,2,4),(-0.606200453641641,-0.30343602424441,
-9.0120313562092E-5),.UNSPECIFIED.);
#243=B_SPLINE_CURVE_WITH_KNOTS('',3,(#10100,#10101,#10102,#10103,#10104,
#10105,#10106,#10107,#10108,#10109,#10110,#10111,#10112,#10113,#10114,#10115,
#10116,#10117,#10118,#10119,#10120,#10121,#10122,#10123,#10124,#10125,#10126,
#10127),.UNSPECIFIED.,.F.,.F.,(4,3,3,3,3,3,3,3,3,4),(-0.152277688086818,
-0.128551334178815,-0.115197577176818,-0.0912856014461669,-0.0781191417238373,
-0.0652765169533013,-0.0414883027365163,-0.0390570310290822,-0.0152653090895913,
0.),.UNSPECIFIED.);
#244=B_SPLINE_CURVE_WITH_KNOTS('',3,(#10129,#10130,#10131,#10132,#10133,
#10134),.UNSPECIFIED.,.F.,.F.,(4,2,4),(-0.60678286609787,-0.303436074842897,
-0.000672492961417026),.UNSPECIFIED.);
#245=B_SPLINE_CURVE_WITH_KNOTS('',3,(#10151,#10152,#10153,#10154),
 .UNSPECIFIED.,.F.,.F.,(4,4),(-9.65082888146972,-7.25285594219682),
 .UNSPECIFIED.);
#246=B_SPLINE_CURVE_WITH_KNOTS('',3,(#10175,#10176,#10177,#10178),
 .UNSPECIFIED.,.F.,.F.,(4,4),(7.25489642332205,7.94751235889625),
 .UNSPECIFIED.);
#247=B_SPLINE_CURVE_WITH_KNOTS('',3,(#10179,#10180,#10181,#10182),
 .UNSPECIFIED.,.F.,.F.,(4,4),(8.17787511801303,9.65708648657758),
 .UNSPECIFIED.);
#248=B_SPLINE_CURVE_WITH_KNOTS('',3,(#10202,#10203,#10204,#10205,#10206,
#10207),.UNSPECIFIED.,.F.,.F.,(4,2,4),(-0.607007797795788,-0.303636495504298,
-0.000571323176327465),.UNSPECIFIED.);
#249=B_SPLINE_CURVE_WITH_KNOTS('',3,(#10209,#10210,#10211,#10212,#10213,
#10214,#10215,#10216,#10217,#10218,#10219,#10220,#10221,#10222,#10223,#10224,
#10225,#10226,#10227,#10228,#10229,#10230,#10231,#10232,#10233,#10234,#10235,
#10236),.UNSPECIFIED.,.F.,.F.,(4,3,3,3,3,3,3,3,3,4),(-0.152184339020145,
-0.128410461444444,-0.115096394428865,-0.0911692948751363,-0.0780261759644403,
-0.0651939085034322,-0.0413932235702045,-0.0389860720679279,-0.0151971168406065,
0.),.UNSPECIFIED.);
#250=B_SPLINE_CURVE_WITH_KNOTS('',3,(#10240,#10241,#10242,#10243,#10244,
#10245,#10246,#10247,#10248,#10249,#10250,#10251,#10252,#10253,#10254,#10255,
#10256,#10257,#10258,#10259,#10260,#10261,#10262,#10263,#10264,#10265,#10266,
#10267),.UNSPECIFIED.,.F.,.F.,(4,3,3,3,3,3,3,3,3,4),(-0.15219777746951,
-0.128424216118147,-0.115318679085322,-0.0915406112613293,-0.0870190514838729,
-0.0784197287877601,-0.0545085386658457,-0.0392329067084975,-0.0154317870320417,
0.),.UNSPECIFIED.);
#251=B_SPLINE_CURVE_WITH_KNOTS('',3,(#10268,#10269,#10270,#10271,#10272,
#10273),.UNSPECIFIED.,.F.,.F.,(4,2,4),(-0.606706256981509,-0.303636876939173,
-0.00026974181288697),.UNSPECIFIED.);
#252=B_SPLINE_CURVE_WITH_KNOTS('',3,(#10291,#10292,#10293,#10294),
 .UNSPECIFIED.,.F.,.F.,(4,4),(0.0112334529114386,0.618489359031386),
 .UNSPECIFIED.);
#253=B_SPLINE_CURVE_WITH_KNOTS('',3,(#10295,#10296,#10297,#10298),
 .UNSPECIFIED.,.F.,.F.,(4,4),(-10.4271318523291,-9.85085636625011),
 .UNSPECIFIED.);
#254=B_SPLINE_CURVE_WITH_KNOTS('',3,(#10321,#10322,#10323,#10324),
 .UNSPECIFIED.,.F.,.F.,(4,4),(9.85750350611301,10.4271318523291),
 .UNSPECIFIED.);
#255=B_SPLINE_CURVE_WITH_KNOTS('',3,(#10328,#10329,#10330,#10331),
 .UNSPECIFIED.,.F.,.F.,(4,4),(0.27539863731415,0.845026983530265),
 .UNSPECIFIED.);
#256=B_SPLINE_CURVE_WITH_KNOTS('',3,(#10349,#10350,#10351,#10352),
 .UNSPECIFIED.,.F.,.F.,(4,4),(-0.851674123393175,-0.27539863731415),
 .UNSPECIFIED.);
#257=B_SPLINE_CURVE_WITH_KNOTS('',3,(#10353,#10354,#10355,#10356),
 .UNSPECIFIED.,.F.,.F.,(4,4),(-0.618489359031386,-0.0112334529114389),
 .UNSPECIFIED.);
#258=B_SPLINE_CURVE_WITH_KNOTS('',3,(#10436,#10437,#10438,#10439),
 .UNSPECIFIED.,.F.,.F.,(4,4),(0.0112755522169305,0.618164468641375),
 .UNSPECIFIED.);
#259=B_SPLINE_CURVE_WITH_KNOTS('',3,(#10460,#10461,#10462,#10463),
 .UNSPECIFIED.,.F.,.F.,(4,4),(-0.618164468641375,-0.0112755522169305),
 .UNSPECIFIED.);
#260=B_SPLINE_CURVE_WITH_KNOTS('',3,(#10549,#10550,#10551,#10552),
 .UNSPECIFIED.,.F.,.F.,(4,4),(5.55111512312578E-17,0.618489359031386),
 .UNSPECIFIED.);
#261=B_SPLINE_CURVE_WITH_KNOTS('',3,(#10553,#10554,#10555,#10556),
 .UNSPECIFIED.,.F.,.F.,(4,4),(-0.618489359031386,-0.00110654915602034),
 .UNSPECIFIED.);
#262=B_SPLINE_CURVE_WITH_KNOTS('',3,(#10592,#10593,#10594,#10595,#10596),
 .UNSPECIFIED.,.F.,.F.,(4,1,4),(-10.4271318523291,-4.63063308449434,-0.283259008618247),
 .UNSPECIFIED.);
#263=B_SPLINE_CURVE_WITH_KNOTS('',3,(#10597,#10598,#10599,#10600,#10601),
 .UNSPECIFIED.,.F.,.F.,(4,1,4),(0.283259011433087,4.63063308449434,10.4271318523291),
 .UNSPECIFIED.);
#264=B_SPLINE_CURVE_WITH_KNOTS('',3,(#10622,#10623,#10624,#10625),
 .UNSPECIFIED.,.F.,.F.,(4,4),(0.000779732613545348,0.618164468641375),
 .UNSPECIFIED.);
#265=B_SPLINE_CURVE_WITH_KNOTS('',3,(#10626,#10627,#10628,#10629),
 .UNSPECIFIED.,.F.,.F.,(4,4),(-0.618164468641375,-4.9439619065339E-17),
 .UNSPECIFIED.);
#266=B_SPLINE_CURVE_WITH_KNOTS('',3,(#10650,#10651,#10652,#10653),
 .UNSPECIFIED.,.F.,.F.,(4,4),(3.0964814046186E-16,0.618164468641375),
 .UNSPECIFIED.);
#267=B_SPLINE_CURVE_WITH_KNOTS('',3,(#10654,#10655,#10656,#10657),
 .UNSPECIFIED.,.F.,.F.,(4,4),(-0.618164468641375,-0.0007797326135453),
 .UNSPECIFIED.);
#268=B_SPLINE_CURVE_WITH_KNOTS('',3,(#10683,#10684,#10685,#10686,#10687),
 .UNSPECIFIED.,.F.,.F.,(4,1,4),(-10.419271481025,-4.62277271319024,-0.27539863731415),
 .UNSPECIFIED.);
#269=B_SPLINE_CURVE_WITH_KNOTS('',3,(#10688,#10689,#10690,#10691,#10692),
 .UNSPECIFIED.,.F.,.F.,(4,1,4),(0.27539863731415,4.62277271319024,10.419271481025),
 .UNSPECIFIED.);
#270=B_SPLINE_CURVE_WITH_KNOTS('',3,(#10713,#10714,#10715,#10716),
 .UNSPECIFIED.,.F.,.F.,(4,4),(0.00110654915602046,0.618489359031386),
 .UNSPECIFIED.);
#271=B_SPLINE_CURVE_WITH_KNOTS('',3,(#10717,#10718,#10719,#10720),
 .UNSPECIFIED.,.F.,.F.,(4,4),(-0.618489359031386,6.93889390390723E-18),
 .UNSPECIFIED.);
#557=SHAPE_REPRESENTATION_RELATIONSHIP('SRR','None',#18628,#566);
#566=ADVANCED_BREP_SHAPE_REPRESENTATION('',(#584),#18574);
#575=STYLED_ITEM('',(#18686),#584);
#584=MANIFOLD_SOLID_BREP('Body1',#6547);
#599=FACE_BOUND('',#1230,.T.);
#600=FACE_BOUND('',#1231,.T.);
#601=FACE_BOUND('',#1232,.T.);
#602=FACE_BOUND('',#1239,.T.);
#603=FACE_BOUND('',#1242,.T.);
#604=FACE_BOUND('',#1253,.T.);
#605=FACE_BOUND('',#1255,.T.);
#606=FACE_BOUND('',#1267,.T.);
#607=FACE_BOUND('',#1288,.T.);
#608=FACE_BOUND('',#1289,.T.);
#609=FACE_BOUND('',#1290,.T.);
#610=FACE_BOUND('',#1325,.T.);
#611=FACE_BOUND('',#1326,.T.);
#612=FACE_BOUND('',#1327,.T.);
#613=FACE_BOUND('',#1328,.T.);
#614=FACE_BOUND('',#1329,.T.);
#615=FACE_BOUND('',#1330,.T.);
#682=PLANE('',#6731);
#683=PLANE('',#6748);
#684=PLANE('',#6753);
#685=PLANE('',#6759);
#686=PLANE('',#6760);
#687=PLANE('',#6761);
#688=PLANE('',#6762);
#689=PLANE('',#6763);
#690=PLANE('',#6764);
#691=PLANE('',#6765);
#692=PLANE('',#6766);
#693=PLANE('',#6768);
#694=PLANE('',#6770);
#695=PLANE('',#6771);
#696=PLANE('',#6772);
#697=PLANE('',#6773);
#698=PLANE('',#6774);
#699=PLANE('',#6775);
#700=PLANE('',#6776);
#701=PLANE('',#6777);
#702=PLANE('',#6778);
#703=PLANE('',#6779);
#704=PLANE('',#6780);
#705=PLANE('',#6784);
#706=PLANE('',#6786);
#707=PLANE('',#6787);
#708=PLANE('',#6788);
#709=PLANE('',#6789);
#710=PLANE('',#6790);
#711=PLANE('',#6791);
#712=PLANE('',#6793);
#713=PLANE('',#6810);
#714=PLANE('',#6829);
#715=PLANE('',#6830);
#716=PLANE('',#6831);
#838=FACE_OUTER_BOUND('',#1223,.T.);
#839=FACE_OUTER_BOUND('',#1224,.T.);
#840=FACE_OUTER_BOUND('',#1225,.T.);
#841=FACE_OUTER_BOUND('',#1226,.T.);
#842=FACE_OUTER_BOUND('',#1227,.T.);
#843=FACE_OUTER_BOUND('',#1228,.T.);
#844=FACE_OUTER_BOUND('',#1229,.T.);
#845=FACE_OUTER_BOUND('',#1233,.T.);
#846=FACE_OUTER_BOUND('',#1234,.T.);
#847=FACE_OUTER_BOUND('',#1235,.T.);
#848=FACE_OUTER_BOUND('',#1236,.T.);
#849=FACE_OUTER_BOUND('',#1237,.T.);
#850=FACE_OUTER_BOUND('',#1238,.T.);
#851=FACE_OUTER_BOUND('',#1240,.T.);
#852=FACE_OUTER_BOUND('',#1241,.T.);
#853=FACE_OUTER_BOUND('',#1243,.T.);
#854=FACE_OUTER_BOUND('',#1244,.T.);
#855=FACE_OUTER_BOUND('',#1245,.T.);
#856=FACE_OUTER_BOUND('',#1246,.T.);
#857=FACE_OUTER_BOUND('',#1247,.T.);
#858=FACE_OUTER_BOUND('',#1248,.T.);
#859=FACE_OUTER_BOUND('',#1249,.T.);
#860=FACE_OUTER_BOUND('',#1250,.T.);
#861=FACE_OUTER_BOUND('',#1251,.T.);
#862=FACE_OUTER_BOUND('',#1252,.T.);
#863=FACE_OUTER_BOUND('',#1254,.T.);
#864=FACE_OUTER_BOUND('',#1256,.T.);
#865=FACE_OUTER_BOUND('',#1257,.T.);
#866=FACE_OUTER_BOUND('',#1258,.T.);
#867=FACE_OUTER_BOUND('',#1259,.T.);
#868=FACE_OUTER_BOUND('',#1260,.T.);
#869=FACE_OUTER_BOUND('',#1261,.T.);
#870=FACE_OUTER_BOUND('',#1262,.T.);
#871=FACE_OUTER_BOUND('',#1263,.T.);
#872=FACE_OUTER_BOUND('',#1264,.T.);
#873=FACE_OUTER_BOUND('',#1265,.T.);
#874=FACE_OUTER_BOUND('',#1266,.T.);
#875=FACE_OUTER_BOUND('',#1268,.T.);
#876=FACE_OUTER_BOUND('',#1269,.T.);
#877=FACE_OUTER_BOUND('',#1270,.T.);
#878=FACE_OUTER_BOUND('',#1271,.T.);
#879=FACE_OUTER_BOUND('',#1272,.T.);
#880=FACE_OUTER_BOUND('',#1273,.T.);
#881=FACE_OUTER_BOUND('',#1274,.T.);
#882=FACE_OUTER_BOUND('',#1275,.T.);
#883=FACE_OUTER_BOUND('',#1276,.T.);
#884=FACE_OUTER_BOUND('',#1277,.T.);
#885=FACE_OUTER_BOUND('',#1278,.T.);
#886=FACE_OUTER_BOUND('',#1279,.T.);
#887=FACE_OUTER_BOUND('',#1280,.T.);
#888=FACE_OUTER_BOUND('',#1281,.T.);
#889=FACE_OUTER_BOUND('',#1282,.T.);
#890=FACE_OUTER_BOUND('',#1283,.T.);
#891=FACE_OUTER_BOUND('',#1284,.T.);
#892=FACE_OUTER_BOUND('',#1285,.T.);
#893=FACE_OUTER_BOUND('',#1286,.T.);
#894=FACE_OUTER_BOUND('',#1287,.T.);
#895=FACE_OUTER_BOUND('',#1291,.T.);
#896=FACE_OUTER_BOUND('',#1292,.T.);
#897=FACE_OUTER_BOUND('',#1293,.T.);
#898=FACE_OUTER_BOUND('',#1294,.T.);
#899=FACE_OUTER_BOUND('',#1295,.T.);
#900=FACE_OUTER_BOUND('',#1296,.T.);
#901=FACE_OUTER_BOUND('',#1297,.T.);
#902=FACE_OUTER_BOUND('',#1298,.T.);
#903=FACE_OUTER_BOUND('',#1299,.T.);
#904=FACE_OUTER_BOUND('',#1300,.T.);
#905=FACE_OUTER_BOUND('',#1301,.T.);
#906=FACE_OUTER_BOUND('',#1302,.T.);
#907=FACE_OUTER_BOUND('',#1303,.T.);
#908=FACE_OUTER_BOUND('',#1304,.T.);
#909=FACE_OUTER_BOUND('',#1305,.T.);
#910=FACE_OUTER_BOUND('',#1306,.T.);
#911=FACE_OUTER_BOUND('',#1307,.T.);
#912=FACE_OUTER_BOUND('',#1308,.T.);
#913=FACE_OUTER_BOUND('',#1309,.T.);
#914=FACE_OUTER_BOUND('',#1310,.T.);
#915=FACE_OUTER_BOUND('',#1311,.T.);
#916=FACE_OUTER_BOUND('',#1312,.T.);
#917=FACE_OUTER_BOUND('',#1313,.T.);
#918=FACE_OUTER_BOUND('',#1314,.T.);
#919=FACE_OUTER_BOUND('',#1315,.T.);
#920=FACE_OUTER_BOUND('',#1316,.T.);
#921=FACE_OUTER_BOUND('',#1317,.T.);
#922=FACE_OUTER_BOUND('',#1318,.T.);
#923=FACE_OUTER_BOUND('',#1319,.T.);
#924=FACE_OUTER_BOUND('',#1320,.T.);
#925=FACE_OUTER_BOUND('',#1321,.T.);
#926=FACE_OUTER_BOUND('',#1322,.T.);
#927=FACE_OUTER_BOUND('',#1323,.T.);
#928=FACE_OUTER_BOUND('',#1324,.T.);
#929=FACE_OUTER_BOUND('',#1331,.T.);
#930=FACE_OUTER_BOUND('',#1332,.T.);
#1223=EDGE_LOOP('',(#4334,#4335));
#1224=EDGE_LOOP('',(#4336,#4337));
#1225=EDGE_LOOP('',(#4338,#4339));
#1226=EDGE_LOOP('',(#4340,#4341));
#1227=EDGE_LOOP('',(#4342,#4343,#4344,#4345,#4346,#4347));
#1228=EDGE_LOOP('',(#4348,#4349,#4350,#4351,#4352,#4353));
#1229=EDGE_LOOP('',(#4354,#4355,#4356,#4357,#4358,#4359,#4360,#4361));
#1230=EDGE_LOOP('',(#4362));
#1231=EDGE_LOOP('',(#4363));
#1232=EDGE_LOOP('',(#4364));
#1233=EDGE_LOOP('',(#4365,#4366,#4367,#4368));
#1234=EDGE_LOOP('',(#4369,#4370,#4371,#4372));
#1235=EDGE_LOOP('',(#4373,#4374,#4375,#4376));
#1236=EDGE_LOOP('',(#4377,#4378,#4379,#4380));
#1237=EDGE_LOOP('',(#4381,#4382,#4383,#4384));
#1238=EDGE_LOOP('',(#4385));
#1239=EDGE_LOOP('',(#4386));
#1240=EDGE_LOOP('',(#4387,#4388,#4389,#4390));
#1241=EDGE_LOOP('',(#4391));
#1242=EDGE_LOOP('',(#4392));
#1243=EDGE_LOOP('',(#4393,#4394,#4395,#4396));
#1244=EDGE_LOOP('',(#4397,#4398,#4399,#4400));
#1245=EDGE_LOOP('',(#4401,#4402,#4403,#4404));
#1246=EDGE_LOOP('',(#4405,#4406,#4407,#4408));
#1247=EDGE_LOOP('',(#4409,#4410,#4411,#4412));
#1248=EDGE_LOOP('',(#4413,#4414,#4415,#4416));
#1249=EDGE_LOOP('',(#4417,#4418,#4419,#4420));
#1250=EDGE_LOOP('',(#4421,#4422,#4423,#4424));
#1251=EDGE_LOOP('',(#4425,#4426,#4427,#4428));
#1252=EDGE_LOOP('',(#4429));
#1253=EDGE_LOOP('',(#4430));
#1254=EDGE_LOOP('',(#4431));
#1255=EDGE_LOOP('',(#4432));
#1256=EDGE_LOOP('',(#4433,#4434,#4435,#4436));
#1257=EDGE_LOOP('',(#4437,#4438,#4439,#4440));
#1258=EDGE_LOOP('',(#4441,#4442,#4443,#4444));
#1259=EDGE_LOOP('',(#4445,#4446,#4447,#4448));
#1260=EDGE_LOOP('',(#4449,#4450,#4451,#4452));
#1261=EDGE_LOOP('',(#4453,#4454,#4455,#4456,#4457,#4458));
#1262=EDGE_LOOP('',(#4459,#4460,#4461,#4462,#4463,#4464,#4465,#4466,#4467,
#4468));
#1263=EDGE_LOOP('',(#4469,#4470,#4471,#4472,#4473,#4474,#4475,#4476,#4477,
#4478));
#1264=EDGE_LOOP('',(#4479,#4480,#4481,#4482,#4483,#4484,#4485,#4486,#4487,
#4488));
#1265=EDGE_LOOP('',(#4489,#4490,#4491,#4492,#4493,#4494,#4495,#4496));
#1266=EDGE_LOOP('',(#4497,#4498,#4499,#4500,#4501,#4502,#4503,#4504,#4505,
#4506,#4507,#4508,#4509,#4510,#4511,#4512,#4513,#4514,#4515,#4516,#4517,
#4518,#4519,#4520,#4521,#4522,#4523,#4524,#4525,#4526,#4527,#4528,#4529,
#4530,#4531,#4532,#4533,#4534,#4535,#4536,#4537,#4538));
#1267=EDGE_LOOP('',(#4539,#4540,#4541,#4542,#4543,#4544));
#1268=EDGE_LOOP('',(#4545,#4546,#4547,#4548));
#1269=EDGE_LOOP('',(#4549,#4550,#4551,#4552));
#1270=EDGE_LOOP('',(#4553,#4554,#4555,#4556,#4557,#4558));
#1271=EDGE_LOOP('',(#4559,#4560,#4561,#4562));
#1272=EDGE_LOOP('',(#4563,#4564,#4565,#4566));
#1273=EDGE_LOOP('',(#4567,#4568,#4569,#4570,#4571,#4572));
#1274=EDGE_LOOP('',(#4573,#4574,#4575,#4576));
#1275=EDGE_LOOP('',(#4577,#4578,#4579,#4580));
#1276=EDGE_LOOP('',(#4581,#4582,#4583,#4584));
#1277=EDGE_LOOP('',(#4585,#4586,#4587,#4588));
#1278=EDGE_LOOP('',(#4589,#4590,#4591,#4592,#4593,#4594,#4595,#4596,#4597,
#4598));
#1279=EDGE_LOOP('',(#4599,#4600,#4601,#4602));
#1280=EDGE_LOOP('',(#4603,#4604,#4605,#4606));
#1281=EDGE_LOOP('',(#4607,#4608,#4609,#4610));
#1282=EDGE_LOOP('',(#4611,#4612,#4613,#4614));
#1283=EDGE_LOOP('',(#4615,#4616,#4617,#4618));
#1284=EDGE_LOOP('',(#4619,#4620,#4621,#4622,#4623,#4624,#4625,#4626,#4627,
#4628));
#1285=EDGE_LOOP('',(#4629,#4630,#4631,#4632));
#1286=EDGE_LOOP('',(#4633,#4634,#4635,#4636,#4637,#4638));
#1287=EDGE_LOOP('',(#4639,#4640,#4641,#4642,#4643,#4644,#4645,#4646));
#1288=EDGE_LOOP('',(#4647));
#1289=EDGE_LOOP('',(#4648));
#1290=EDGE_LOOP('',(#4649));
#1291=EDGE_LOOP('',(#4650,#4651,#4652,#4653));
#1292=EDGE_LOOP('',(#4654,#4655,#4656,#4657,#4658,#4659,#4660,#4661,#4662,
#4663));
#1293=EDGE_LOOP('',(#4664,#4665,#4666,#4667));
#1294=EDGE_LOOP('',(#4668,#4669,#4670,#4671));
#1295=EDGE_LOOP('',(#4672,#4673,#4674,#4675));
#1296=EDGE_LOOP('',(#4676,#4677,#4678,#4679));
#1297=EDGE_LOOP('',(#4680,#4681,#4682,#4683));
#1298=EDGE_LOOP('',(#4684,#4685,#4686));
#1299=EDGE_LOOP('',(#4687,#4688,#4689));
#1300=EDGE_LOOP('',(#4690,#4691,#4692));
#1301=EDGE_LOOP('',(#4693,#4694,#4695,#4696));
#1302=EDGE_LOOP('',(#4697,#4698,#4699,#4700));
#1303=EDGE_LOOP('',(#4701,#4702,#4703));
#1304=EDGE_LOOP('',(#4704,#4705,#4706,#4707));
#1305=EDGE_LOOP('',(#4708,#4709,#4710,#4711));
#1306=EDGE_LOOP('',(#4712,#4713,#4714,#4715));
#1307=EDGE_LOOP('',(#4716,#4717,#4718,#4719));
#1308=EDGE_LOOP('',(#4720,#4721,#4722,#4723));
#1309=EDGE_LOOP('',(#4724,#4725,#4726,#4727));
#1310=EDGE_LOOP('',(#4728,#4729,#4730));
#1311=EDGE_LOOP('',(#4731,#4732,#4733));
#1312=EDGE_LOOP('',(#4734,#4735,#4736));
#1313=EDGE_LOOP('',(#4737,#4738,#4739,#4740));
#1314=EDGE_LOOP('',(#4741,#4742,#4743,#4744));
#1315=EDGE_LOOP('',(#4745,#4746,#4747));
#1316=EDGE_LOOP('',(#4748,#4749,#4750,#4751));
#1317=EDGE_LOOP('',(#4752,#4753,#4754,#4755));
#1318=EDGE_LOOP('',(#4756,#4757,#4758,#4759));
#1319=EDGE_LOOP('',(#4760,#4761,#4762,#4763));
#1320=EDGE_LOOP('',(#4764,#4765,#4766,#4767));
#1321=EDGE_LOOP('',(#4768,#4769,#4770,#4771));
#1322=EDGE_LOOP('',(#4772,#4773,#4774,#4775));
#1323=EDGE_LOOP('',(#4776,#4777,#4778,#4779,#4780,#4781,#4782,#4783));
#1324=EDGE_LOOP('',(#4784,#4785,#4786,#4787));
#1325=EDGE_LOOP('',(#4788));
#1326=EDGE_LOOP('',(#4789));
#1327=EDGE_LOOP('',(#4790));
#1328=EDGE_LOOP('',(#4791));
#1329=EDGE_LOOP('',(#4792));
#1330=EDGE_LOOP('',(#4793));
#1331=EDGE_LOOP('',(#4794,#4795,#4796,#4797));
#1332=EDGE_LOOP('',(#4798,#4799,#4800,#4801));
#1684=LINE('',#9006,#2091);
#1685=LINE('',#9008,#2092);
#1686=LINE('',#9022,#2093);
#1687=LINE('',#9027,#2094);
#1688=LINE('',#9033,#2095);
#1689=LINE('',#9038,#2096);
#1690=LINE('',#9043,#2097);
#1691=LINE('',#9052,#2098);
#1692=LINE('',#9059,#2099);
#1693=LINE('',#9063,#2100);
#1694=LINE('',#9068,#2101);
#1695=LINE('',#9070,#2102);
#1696=LINE('',#9072,#2103);
#1697=LINE('',#9073,#2104);
#1698=LINE('',#9077,#2105);
#1699=LINE('',#9079,#2106);
#1700=LINE('',#9081,#2107);
#1701=LINE('',#9082,#2108);
#1702=LINE('',#9086,#2109);
#1703=LINE('',#9088,#2110);
#1704=LINE('',#9090,#2111);
#1705=LINE('',#9091,#2112);
#1706=LINE('',#9095,#2113);
#1707=LINE('',#9097,#2114);
#1708=LINE('',#9099,#2115);
#1709=LINE('',#9100,#2116);
#1710=LINE('',#9104,#2117);
#1711=LINE('',#9106,#2118);
#1712=LINE('',#9108,#2119);
#1713=LINE('',#9109,#2120);
#1714=LINE('',#9113,#2121);
#1715=LINE('',#9115,#2122);
#1716=LINE('',#9117,#2123);
#1717=LINE('',#9118,#2124);
#1718=LINE('',#9122,#2125);
#1719=LINE('',#9124,#2126);
#1720=LINE('',#9126,#2127);
#1721=LINE('',#9127,#2128);
#1722=LINE('',#9135,#2129);
#1723=LINE('',#9136,#2130);
#1724=LINE('',#9138,#2131);
#1725=LINE('',#9139,#2132);
#1726=LINE('',#9141,#2133);
#1727=LINE('',#9142,#2134);
#1728=LINE('',#9145,#2135);
#1729=LINE('',#9147,#2136);
#1730=LINE('',#9148,#2137);
#1731=LINE('',#9151,#2138);
#1732=LINE('',#9153,#2139);
#1733=LINE('',#9154,#2140);
#1734=LINE('',#9158,#2141);
#1735=LINE('',#9202,#2142);
#1736=LINE('',#9245,#2143);
#1737=LINE('',#9248,#2144);
#1738=LINE('',#9286,#2145);
#1739=LINE('',#9323,#2146);
#1740=LINE('',#9326,#2147);
#1741=LINE('',#9334,#2148);
#1742=LINE('',#9371,#2149);
#1743=LINE('',#9374,#2150);
#1744=LINE('',#9381,#2151);
#1745=LINE('',#9387,#2152);
#1746=LINE('',#9398,#2153);
#1747=LINE('',#9407,#2154);
#1748=LINE('',#9413,#2155);
#1749=LINE('',#9448,#2156);
#1750=LINE('',#9519,#2157);
#1751=LINE('',#9589,#2158);
#1752=LINE('',#9621,#2159);
#1753=LINE('',#9627,#2160);
#1754=LINE('',#9636,#2161);
#1755=LINE('',#9673,#2162);
#1756=LINE('',#9708,#2163);
#1757=LINE('',#9710,#2164);
#1758=LINE('',#9714,#2165);
#1759=LINE('',#9760,#2166);
#1760=LINE('',#9886,#2167);
#1761=LINE('',#9966,#2168);
#1762=LINE('',#10128,#2169);
#1763=LINE('',#10238,#2170);
#1764=LINE('',#10327,#2171);
#1765=LINE('',#10415,#2172);
#1766=LINE('',#10527,#2173);
#1767=LINE('',#10528,#2174);
#1768=LINE('',#10565,#2175);
#1769=LINE('',#10566,#2176);
#2091=VECTOR('',#7367,1.);
#2092=VECTOR('',#7368,1.);
#2093=VECTOR('',#7379,0.15);
#2094=VECTOR('',#7384,0.15);
#2095=VECTOR('',#7391,0.15);
#2096=VECTOR('',#7398,0.15);
#2097=VECTOR('',#7403,0.3);
#2098=VECTOR('',#7414,0.3);
#2099=VECTOR('',#7423,0.17);
#2100=VECTOR('',#7428,0.17);
#2101=VECTOR('',#7433,1.);
#2102=VECTOR('',#7434,1.);
#2103=VECTOR('',#7435,1.);
#2104=VECTOR('',#7436,1.);
#2105=VECTOR('',#7439,1.);
#2106=VECTOR('',#7440,1.);
#2107=VECTOR('',#7441,1.);
#2108=VECTOR('',#7442,1.);
#2109=VECTOR('',#7445,1.);
#2110=VECTOR('',#7446,1.);
#2111=VECTOR('',#7447,1.);
#2112=VECTOR('',#7448,1.);
#2113=VECTOR('',#7451,1.);
#2114=VECTOR('',#7452,1.);
#2115=VECTOR('',#7453,1.);
#2116=VECTOR('',#7454,1.);
#2117=VECTOR('',#7457,1.);
#2118=VECTOR('',#7458,1.);
#2119=VECTOR('',#7459,1.);
#2120=VECTOR('',#7460,1.);
#2121=VECTOR('',#7463,1.);
#2122=VECTOR('',#7464,1.);
#2123=VECTOR('',#7465,1.);
#2124=VECTOR('',#7466,1.);
#2125=VECTOR('',#7469,1.);
#2126=VECTOR('',#7470,1.);
#2127=VECTOR('',#7471,1.);
#2128=VECTOR('',#7472,1.);
#2129=VECTOR('',#7483,1.);
#2130=VECTOR('',#7484,1.);
#2131=VECTOR('',#7487,1.);
#2132=VECTOR('',#7488,1.);
#2133=VECTOR('',#7491,1.);
#2134=VECTOR('',#7492,1.);
#2135=VECTOR('',#7495,1.);
#2136=VECTOR('',#7496,1.);
#2137=VECTOR('',#7497,1.);
#2138=VECTOR('',#7500,1.);
#2139=VECTOR('',#7501,1.);
#2140=VECTOR('',#7502,1.);
#2141=VECTOR('',#7505,1.);
#2142=VECTOR('',#7508,1.);
#2143=VECTOR('',#7509,1.);
#2144=VECTOR('',#7512,1.);
#2145=VECTOR('',#7513,1.);
#2146=VECTOR('',#7514,1.);
#2147=VECTOR('',#7517,1.);
#2148=VECTOR('',#7518,1.);
#2149=VECTOR('',#7519,1.);
#2150=VECTOR('',#7522,1.);
#2151=VECTOR('',#7523,1.);
#2152=VECTOR('',#7524,1.);
#2153=VECTOR('',#7527,1.);
#2154=VECTOR('',#7528,1.);
#2155=VECTOR('',#7529,1.);
#2156=VECTOR('',#7530,1.);
#2157=VECTOR('',#7531,1.);
#2158=VECTOR('',#7532,1.);
#2159=VECTOR('',#7533,1.);
#2160=VECTOR('',#7534,1.);
#2161=VECTOR('',#7535,1.);
#2162=VECTOR('',#7536,1.);
#2163=VECTOR('',#7537,1.);
#2164=VECTOR('',#7540,0.4);
#2165=VECTOR('',#7545,0.4);
#2166=VECTOR('',#7548,1.);
#2167=VECTOR('',#7553,1.);
#2168=VECTOR('',#7556,1.);
#2169=VECTOR('',#7561,1.);
#2170=VECTOR('',#7566,1.);
#2171=VECTOR('',#7571,1.);
#2172=VECTOR('',#7604,1.);
#2173=VECTOR('',#7633,1.);
#2174=VECTOR('',#7634,1.);
#2175=VECTOR('',#7645,1.);
#2176=VECTOR('',#7646,1.);
#2445=CIRCLE('',#6724,0.25);
#2446=CIRCLE('',#6726,0.25);
#2447=CIRCLE('',#6728,0.25);
#2448=CIRCLE('',#6730,0.25);
#2449=CIRCLE('',#6732,0.15);
#2450=CIRCLE('',#6733,0.15);
#2451=CIRCLE('',#6734,0.4);
#2452=CIRCLE('',#6736,0.15);
#2453=CIRCLE('',#6738,0.15);
#2454=CIRCLE('',#6739,0.15);
#2455=CIRCLE('',#6741,0.15);
#2456=CIRCLE('',#6742,0.15);
#2457=CIRCLE('',#6744,0.15);
#2458=CIRCLE('',#6746,0.3);
#2459=CIRCLE('',#6747,0.3);
#2460=CIRCLE('',#6749,0.17);
#2461=CIRCLE('',#6751,0.3);
#2462=CIRCLE('',#6752,0.3);
#2463=CIRCLE('',#6754,0.17);
#2464=CIRCLE('',#6756,0.17);
#2465=CIRCLE('',#6758,0.17);
#2466=CIRCLE('',#6767,0.4);
#2467=CIRCLE('',#6769,0.4);
#2468=CIRCLE('',#6783,0.4);
#2469=CIRCLE('',#6785,0.1);
#2470=CIRCLE('',#6792,0.0999999999999995);
#2471=CIRCLE('',#6794,0.1);
#2472=CIRCLE('',#6796,0.1);
#2473=CIRCLE('',#6797,0.1);
#2474=CIRCLE('',#6799,0.0999999999999999);
#2475=CIRCLE('',#6800,0.0999999999999998);
#2476=CIRCLE('',#6801,0.0999999999999998);
#2477=CIRCLE('',#6803,0.0999999999999994);
#2478=CIRCLE('',#6804,0.0999999999999993);
#2479=CIRCLE('',#6807,0.0999999999999999);
#2480=CIRCLE('',#6808,0.1);
#2481=CIRCLE('',#6812,0.3);
#2482=CIRCLE('',#6813,0.3);
#2483=CIRCLE('',#6814,0.3);
#2484=CIRCLE('',#6816,0.3);
#2485=CIRCLE('',#6817,0.3);
#2486=CIRCLE('',#6818,0.3);
#2487=CIRCLE('',#6820,0.3);
#2488=CIRCLE('',#6821,0.299999999999999);
#2489=CIRCLE('',#6822,0.3);
#2490=CIRCLE('',#6825,0.3);
#2491=CIRCLE('',#6826,0.3);
#2492=CIRCLE('',#6827,0.3);
#2645=VERTEX_POINT('',#8713);
#2646=VERTEX_POINT('',#8714);
#2647=VERTEX_POINT('',#8741);
#2648=VERTEX_POINT('',#8742);
#2649=VERTEX_POINT('',#8765);
#2650=VERTEX_POINT('',#8766);
#2651=VERTEX_POINT('',#8789);
#2652=VERTEX_POINT('',#8790);
#2653=VERTEX_POINT('',#8836);
#2654=VERTEX_POINT('',#8841);
#2655=VERTEX_POINT('',#8870);
#2656=VERTEX_POINT('',#8875);
#2657=VERTEX_POINT('',#8928);
#2658=VERTEX_POINT('',#8933);
#2659=VERTEX_POINT('',#8962);
#2660=VERTEX_POINT('',#8967);
#2661=VERTEX_POINT('',#9001);
#2662=VERTEX_POINT('',#9007);
#2663=VERTEX_POINT('',#9013);
#2664=VERTEX_POINT('',#9015);
#2665=VERTEX_POINT('',#9017);
#2666=VERTEX_POINT('',#9020);
#2667=VERTEX_POINT('',#9024);
#2668=VERTEX_POINT('',#9026);
#2669=VERTEX_POINT('',#9030);
#2670=VERTEX_POINT('',#9032);
#2671=VERTEX_POINT('',#9036);
#2672=VERTEX_POINT('',#9040);
#2673=VERTEX_POINT('',#9042);
#2674=VERTEX_POINT('',#9046);
#2675=VERTEX_POINT('',#9049);
#2676=VERTEX_POINT('',#9051);
#2677=VERTEX_POINT('',#9055);
#2678=VERTEX_POINT('',#9058);
#2679=VERTEX_POINT('',#9062);
#2680=VERTEX_POINT('',#9066);
#2681=VERTEX_POINT('',#9067);
#2682=VERTEX_POINT('',#9069);
#2683=VERTEX_POINT('',#9071);
#2684=VERTEX_POINT('',#9075);
#2685=VERTEX_POINT('',#9076);
#2686=VERTEX_POINT('',#9078);
#2687=VERTEX_POINT('',#9080);
#2688=VERTEX_POINT('',#9084);
#2689=VERTEX_POINT('',#9085);
#2690=VERTEX_POINT('',#9087);
#2691=VERTEX_POINT('',#9089);
#2692=VERTEX_POINT('',#9093);
#2693=VERTEX_POINT('',#9094);
#2694=VERTEX_POINT('',#9096);
#2695=VERTEX_POINT('',#9098);
#2696=VERTEX_POINT('',#9102);
#2697=VERTEX_POINT('',#9103);
#2698=VERTEX_POINT('',#9105);
#2699=VERTEX_POINT('',#9107);
#2700=VERTEX_POINT('',#9111);
#2701=VERTEX_POINT('',#9112);
#2702=VERTEX_POINT('',#9114);
#2703=VERTEX_POINT('',#9116);
#2704=VERTEX_POINT('',#9120);
#2705=VERTEX_POINT('',#9121);
#2706=VERTEX_POINT('',#9123);
#2707=VERTEX_POINT('',#9125);
#2708=VERTEX_POINT('',#9129);
#2709=VERTEX_POINT('',#9132);
#2710=VERTEX_POINT('',#9144);
#2711=VERTEX_POINT('',#9146);
#2712=VERTEX_POINT('',#9150);
#2713=VERTEX_POINT('',#9152);
#2714=VERTEX_POINT('',#9156);
#2715=VERTEX_POINT('',#9157);
#2716=VERTEX_POINT('',#9159);
#2717=VERTEX_POINT('',#9201);
#2718=VERTEX_POINT('',#9209);
#2719=VERTEX_POINT('',#9238);
#2720=VERTEX_POINT('',#9247);
#2721=VERTEX_POINT('',#9249);
#2722=VERTEX_POINT('',#9256);
#2723=VERTEX_POINT('',#9285);
#2724=VERTEX_POINT('',#9287);
#2725=VERTEX_POINT('',#9316);
#2726=VERTEX_POINT('',#9325);
#2727=VERTEX_POINT('',#9333);
#2728=VERTEX_POINT('',#9335);
#2729=VERTEX_POINT('',#9364);
#2730=VERTEX_POINT('',#9373);
#2731=VERTEX_POINT('',#9375);
#2732=VERTEX_POINT('',#9380);
#2733=VERTEX_POINT('',#9382);
#2734=VERTEX_POINT('',#9397);
#2735=VERTEX_POINT('',#9406);
#2736=VERTEX_POINT('',#9412);
#2737=VERTEX_POINT('',#9414);
#2738=VERTEX_POINT('',#9447);
#2739=VERTEX_POINT('',#9449);
#2740=VERTEX_POINT('',#9481);
#2741=VERTEX_POINT('',#9486);
#2742=VERTEX_POINT('',#9518);
#2743=VERTEX_POINT('',#9520);
#2744=VERTEX_POINT('',#9552);
#2745=VERTEX_POINT('',#9557);
#2746=VERTEX_POINT('',#9590);
#2747=VERTEX_POINT('',#9616);
#2748=VERTEX_POINT('',#9622);
#2749=VERTEX_POINT('',#9628);
#2750=VERTEX_POINT('',#9637);
#2751=VERTEX_POINT('',#9638);
#2752=VERTEX_POINT('',#9643);
#2753=VERTEX_POINT('',#9672);
#2754=VERTEX_POINT('',#9674);
#2755=VERTEX_POINT('',#9703);
#2756=VERTEX_POINT('',#9712);
#2757=VERTEX_POINT('',#9716);
#2758=VERTEX_POINT('',#9723);
#2759=VERTEX_POINT('',#9730);
#2760=VERTEX_POINT('',#9759);
#2761=VERTEX_POINT('',#9825);
#2762=VERTEX_POINT('',#9874);
#2763=VERTEX_POINT('',#9881);
#2764=VERTEX_POINT('',#9919);
#2765=VERTEX_POINT('',#9929);
#2766=VERTEX_POINT('',#9936);
#2767=VERTEX_POINT('',#9965);
#2768=VERTEX_POINT('',#9967);
#2769=VERTEX_POINT('',#10092);
#2770=VERTEX_POINT('',#10099);
#2771=VERTEX_POINT('',#10201);
#2772=VERTEX_POINT('',#10208);
#2773=VERTEX_POINT('',#10237);
#2774=VERTEX_POINT('',#10239);
#2775=VERTEX_POINT('',#10290);
#2776=VERTEX_POINT('',#10319);
#2777=VERTEX_POINT('',#10326);
#2778=VERTEX_POINT('',#10348);
#2779=VERTEX_POINT('',#10383);
#2780=VERTEX_POINT('',#10411);
#2781=VERTEX_POINT('',#10506);
#2782=VERTEX_POINT('',#10507);
#2783=VERTEX_POINT('',#10509);
#2784=VERTEX_POINT('',#10513);
#2785=VERTEX_POINT('',#10514);
#2786=VERTEX_POINT('',#10516);
#2787=VERTEX_POINT('',#10520);
#2788=VERTEX_POINT('',#10521);
#2789=VERTEX_POINT('',#10523);
#2790=VERTEX_POINT('',#10558);
#2791=VERTEX_POINT('',#10559);
#2792=VERTEX_POINT('',#10561);
#3290=EDGE_CURVE('',#2645,#2646,#172,.T.);
#3291=EDGE_CURVE('',#2645,#2646,#2445,.T.);
#3292=EDGE_CURVE('',#2647,#2648,#173,.T.);
#3293=EDGE_CURVE('',#2647,#2648,#2446,.T.);
#3294=EDGE_CURVE('',#2649,#2650,#174,.T.);
#3295=EDGE_CURVE('',#2649,#2650,#2447,.T.);
#3296=EDGE_CURVE('',#2651,#2652,#175,.T.);
#3297=EDGE_CURVE('',#2651,#2652,#2448,.T.);
#3298=EDGE_CURVE('',#2653,#2648,#176,.T.);
#3299=EDGE_CURVE('',#2653,#2654,#177,.T.);
#3300=EDGE_CURVE('',#2655,#2654,#178,.T.);
#3301=EDGE_CURVE('',#2655,#2656,#179,.T.);
#3302=EDGE_CURVE('',#2647,#2656,#180,.T.);
#3303=EDGE_CURVE('',#2657,#2652,#181,.T.);
#3304=EDGE_CURVE('',#2657,#2658,#182,.T.);
#3305=EDGE_CURVE('',#2659,#2658,#183,.T.);
#3306=EDGE_CURVE('',#2659,#2660,#184,.T.);
#3307=EDGE_CURVE('',#2651,#2660,#185,.T.);
#3308=EDGE_CURVE('',#2645,#2661,#186,.T.);
#3309=EDGE_CURVE('',#2661,#2657,#1684,.T.);
#3310=EDGE_CURVE('',#2660,#2662,#1685,.T.);
#3311=EDGE_CURVE('',#2662,#2646,#187,.T.);
#3312=EDGE_CURVE('',#2663,#2663,#2449,.T.);
#3313=EDGE_CURVE('',#2664,#2664,#2450,.T.);
#3314=EDGE_CURVE('',#2665,#2665,#2451,.T.);
#3315=EDGE_CURVE('',#2666,#2666,#2452,.T.);
#3316=EDGE_CURVE('',#2666,#2663,#1686,.T.);
#3317=EDGE_CURVE('',#2667,#2667,#2453,.T.);
#3318=EDGE_CURVE('',#2667,#2668,#1687,.T.);
#3319=EDGE_CURVE('',#2668,#2668,#2454,.T.);
#3320=EDGE_CURVE('',#2669,#2669,#2455,.T.);
#3321=EDGE_CURVE('',#2669,#2670,#1688,.T.);
#3322=EDGE_CURVE('',#2670,#2670,#2456,.T.);
#3323=EDGE_CURVE('',#2671,#2671,#2457,.T.);
#3324=EDGE_CURVE('',#2671,#2664,#1689,.T.);
#3325=EDGE_CURVE('',#2672,#2672,#2458,.T.);
#3326=EDGE_CURVE('',#2672,#2673,#1690,.T.);
#3327=EDGE_CURVE('',#2673,#2673,#2459,.T.);
#3328=EDGE_CURVE('',#2674,#2674,#2460,.T.);
#3329=EDGE_CURVE('',#2675,#2675,#2461,.T.);
#3330=EDGE_CURVE('',#2675,#2676,#1691,.T.);
#3331=EDGE_CURVE('',#2676,#2676,#2462,.T.);
#3332=EDGE_CURVE('',#2677,#2677,#2463,.T.);
#3333=EDGE_CURVE('',#2674,#2678,#1692,.T.);
#3334=EDGE_CURVE('',#2678,#2678,#2464,.T.);
#3335=EDGE_CURVE('',#2677,#2679,#1693,.T.);
#3336=EDGE_CURVE('',#2679,#2679,#2465,.T.);
#3337=EDGE_CURVE('',#2680,#2681,#1694,.T.);
#3338=EDGE_CURVE('',#2682,#2680,#1695,.T.);
#3339=EDGE_CURVE('',#2683,#2682,#1696,.T.);
#3340=EDGE_CURVE('',#2683,#2681,#1697,.T.);
#3341=EDGE_CURVE('',#2684,#2685,#1698,.T.);
#3342=EDGE_CURVE('',#2684,#2686,#1699,.T.);
#3343=EDGE_CURVE('',#2687,#2686,#1700,.T.);
#3344=EDGE_CURVE('',#2685,#2687,#1701,.T.);
#3345=EDGE_CURVE('',#2688,#2689,#1702,.T.);
#3346=EDGE_CURVE('',#2688,#2690,#1703,.T.);
#3347=EDGE_CURVE('',#2691,#2690,#1704,.T.);
#3348=EDGE_CURVE('',#2689,#2691,#1705,.T.);
#3349=EDGE_CURVE('',#2692,#2693,#1706,.T.);
#3350=EDGE_CURVE('',#2692,#2694,#1707,.T.);
#3351=EDGE_CURVE('',#2695,#2694,#1708,.T.);
#3352=EDGE_CURVE('',#2693,#2695,#1709,.T.);
#3353=EDGE_CURVE('',#2696,#2697,#1710,.T.);
#3354=EDGE_CURVE('',#2696,#2698,#1711,.T.);
#3355=EDGE_CURVE('',#2699,#2698,#1712,.T.);
#3356=EDGE_CURVE('',#2697,#2699,#1713,.T.);
#3357=EDGE_CURVE('',#2700,#2701,#1714,.T.);
#3358=EDGE_CURVE('',#2702,#2700,#1715,.T.);
#3359=EDGE_CURVE('',#2703,#2702,#1716,.T.);
#3360=EDGE_CURVE('',#2703,#2701,#1717,.T.);
#3361=EDGE_CURVE('',#2704,#2705,#1718,.T.);
#3362=EDGE_CURVE('',#2706,#2704,#1719,.T.);
#3363=EDGE_CURVE('',#2707,#2706,#1720,.T.);
#3364=EDGE_CURVE('',#2707,#2705,#1721,.T.);
#3365=EDGE_CURVE('',#2708,#2708,#2466,.T.);
#3366=EDGE_CURVE('',#2709,#2709,#2467,.T.);
#3367=EDGE_CURVE('',#2681,#2696,#1722,.T.);
#3368=EDGE_CURVE('',#2698,#2683,#1723,.T.);
#3369=EDGE_CURVE('',#2701,#2684,#1724,.T.);
#3370=EDGE_CURVE('',#2686,#2703,#1725,.T.);
#3371=EDGE_CURVE('',#2705,#2688,#1726,.T.);
#3372=EDGE_CURVE('',#2690,#2707,#1727,.T.);
#3373=EDGE_CURVE('',#2710,#2692,#1728,.T.);
#3374=EDGE_CURVE('',#2711,#2710,#1729,.T.);
#3375=EDGE_CURVE('',#2694,#2711,#1730,.T.);
#3376=EDGE_CURVE('',#2712,#2710,#1731,.T.);
#3377=EDGE_CURVE('',#2713,#2712,#1732,.T.);
#3378=EDGE_CURVE('',#2711,#2713,#1733,.T.);
#3379=EDGE_CURVE('',#2714,#2715,#1734,.T.);
#3380=EDGE_CURVE('',#2716,#2715,#188,.T.);
#3381=EDGE_CURVE('',#2662,#2716,#189,.T.);
#3382=EDGE_CURVE('',#2714,#2659,#190,.T.);
#3383=EDGE_CURVE('',#2713,#2717,#1735,.T.);
#3384=EDGE_CURVE('',#2658,#2717,#191,.T.);
#3385=EDGE_CURVE('',#2718,#2661,#192,.T.);
#3386=EDGE_CURVE('',#2719,#2718,#193,.T.);
#3387=EDGE_CURVE('',#2719,#2695,#1736,.T.);
#3388=EDGE_CURVE('',#2706,#2720,#1737,.T.);
#3389=EDGE_CURVE('',#2721,#2720,#194,.T.);
#3390=EDGE_CURVE('',#2722,#2721,#195,.T.);
#3391=EDGE_CURVE('',#2723,#2722,#1738,.T.);
#3392=EDGE_CURVE('',#2724,#2723,#196,.T.);
#3393=EDGE_CURVE('',#2725,#2724,#197,.T.);
#3394=EDGE_CURVE('',#2725,#2691,#1739,.T.);
#3395=EDGE_CURVE('',#2702,#2726,#1740,.T.);
#3396=EDGE_CURVE('',#2654,#2726,#198,.T.);
#3397=EDGE_CURVE('',#2727,#2653,#1741,.T.);
#3398=EDGE_CURVE('',#2728,#2727,#199,.T.);
#3399=EDGE_CURVE('',#2729,#2728,#200,.T.);
#3400=EDGE_CURVE('',#2729,#2687,#1742,.T.);
#3401=EDGE_CURVE('',#2730,#2697,#1743,.T.);
#3402=EDGE_CURVE('',#2730,#2731,#201,.T.);
#3403=EDGE_CURVE('',#2731,#2732,#1744,.T.);
#3404=EDGE_CURVE('',#2732,#2733,#202,.T.);
#3405=EDGE_CURVE('',#2680,#2733,#1745,.T.);
#3406=EDGE_CURVE('',#2719,#2715,#203,.T.);
#3407=EDGE_CURVE('',#2714,#2717,#204,.T.);
#3408=EDGE_CURVE('',#2734,#2712,#1746,.T.);
#3409=EDGE_CURVE('',#2734,#2720,#205,.T.);
#3410=EDGE_CURVE('',#2735,#2704,#1747,.T.);
#3411=EDGE_CURVE('',#2735,#2726,#206,.T.);
#3412=EDGE_CURVE('',#2736,#2700,#1748,.T.);
#3413=EDGE_CURVE('',#2736,#2737,#207,.T.);
#3414=EDGE_CURVE('',#2737,#2730,#208,.T.);
#3415=EDGE_CURVE('',#2699,#2738,#1749,.T.);
#3416=EDGE_CURVE('',#2739,#2738,#209,.T.);
#3417=EDGE_CURVE('',#2739,#2740,#210,.T.);
#3418=EDGE_CURVE('',#2741,#2740,#211,.T.);
#3419=EDGE_CURVE('',#2741,#2742,#1750,.T.);
#3420=EDGE_CURVE('',#2743,#2742,#212,.T.);
#3421=EDGE_CURVE('',#2743,#2744,#213,.T.);
#3422=EDGE_CURVE('',#2745,#2744,#214,.T.);
#3423=EDGE_CURVE('',#2745,#2682,#1751,.T.);
#3424=EDGE_CURVE('',#2733,#2746,#215,.T.);
#3425=EDGE_CURVE('',#2746,#2747,#216,.T.);
#3426=EDGE_CURVE('',#2685,#2747,#1752,.T.);
#3427=EDGE_CURVE('',#2729,#2748,#217,.T.);
#3428=EDGE_CURVE('',#2689,#2748,#1753,.T.);
#3429=EDGE_CURVE('',#2725,#2749,#218,.T.);
#3430=EDGE_CURVE('',#2693,#2749,#1754,.T.);
#3431=EDGE_CURVE('',#2750,#2751,#219,.T.);
#3432=EDGE_CURVE('',#2751,#2752,#220,.T.);
#3433=EDGE_CURVE('',#2752,#2753,#1755,.T.);
#3434=EDGE_CURVE('',#2753,#2754,#221,.T.);
#3435=EDGE_CURVE('',#2754,#2755,#222,.T.);
#3436=EDGE_CURVE('',#2750,#2755,#1756,.T.);
#3437=EDGE_CURVE('',#2665,#2709,#1757,.T.);
#3438=EDGE_CURVE('',#2756,#2756,#2468,.T.);
#3439=EDGE_CURVE('',#2756,#2708,#1758,.T.);
#3440=EDGE_CURVE('',#2750,#2757,#223,.T.);
#3441=EDGE_CURVE('',#2758,#2755,#224,.T.);
#3442=EDGE_CURVE('',#2759,#2758,#225,.T.);
#3443=EDGE_CURVE('',#2760,#2759,#1759,.T.);
#3444=EDGE_CURVE('',#2757,#2760,#226,.T.);
#3445=EDGE_CURVE('',#2718,#2716,#227,.T.);
#3446=EDGE_CURVE('',#2757,#2761,#228,.T.);
#3447=EDGE_CURVE('',#2761,#2751,#229,.T.);
#3448=EDGE_CURVE('',#2762,#2760,#230,.T.);
#3449=EDGE_CURVE('',#2761,#2762,#2469,.F.);
#3450=EDGE_CURVE('',#2759,#2763,#231,.T.);
#3451=EDGE_CURVE('',#2763,#2762,#1760,.T.);
#3452=EDGE_CURVE('',#2754,#2764,#232,.T.);
#3453=EDGE_CURVE('',#2764,#2758,#233,.T.);
#3454=EDGE_CURVE('',#2765,#2749,#234,.T.);
#3455=EDGE_CURVE('',#2766,#2765,#235,.T.);
#3456=EDGE_CURVE('',#2767,#2766,#1761,.T.);
#3457=EDGE_CURVE('',#2768,#2767,#236,.T.);
#3458=EDGE_CURVE('',#2734,#2768,#237,.T.);
#3459=EDGE_CURVE('',#2724,#2765,#238,.T.);
#3460=EDGE_CURVE('',#2766,#2723,#239,.T.);
#3461=EDGE_CURVE('',#2722,#2767,#240,.T.);
#3462=EDGE_CURVE('',#2768,#2721,#241,.T.);
#3463=EDGE_CURVE('',#2769,#2748,#242,.T.);
#3464=EDGE_CURVE('',#2770,#2769,#243,.T.);
#3465=EDGE_CURVE('',#2656,#2770,#1762,.T.);
#3466=EDGE_CURVE('',#2735,#2655,#244,.T.);
#3467=EDGE_CURVE('',#2728,#2769,#245,.T.);
#3468=EDGE_CURVE('',#2770,#2650,#246,.T.);
#3469=EDGE_CURVE('',#2649,#2727,#247,.T.);
#3470=EDGE_CURVE('',#2771,#2747,#248,.T.);
#3471=EDGE_CURVE('',#2772,#2771,#249,.T.);
#3472=EDGE_CURVE('',#2773,#2772,#1763,.T.);
#3473=EDGE_CURVE('',#2774,#2773,#250,.T.);
#3474=EDGE_CURVE('',#2736,#2774,#251,.T.);
#3475=EDGE_CURVE('',#2746,#2775,#252,.T.);
#3476=EDGE_CURVE('',#2775,#2771,#253,.T.);
#3477=EDGE_CURVE('',#2776,#2775,#2470,.F.);
#3478=EDGE_CURVE('',#2772,#2776,#254,.T.);
#3479=EDGE_CURVE('',#2776,#2777,#1764,.T.);
#3480=EDGE_CURVE('',#2777,#2773,#255,.T.);
#3481=EDGE_CURVE('',#2774,#2778,#256,.T.);
#3482=EDGE_CURVE('',#2778,#2737,#257,.T.);
#3483=EDGE_CURVE('',#2778,#2777,#2471,.F.);
#3484=EDGE_CURVE('',#2777,#2731,#2472,.F.);
#3485=EDGE_CURVE('',#2731,#2778,#2473,.F.);
#3486=EDGE_CURVE('',#2763,#2764,#2474,.F.);
#3487=EDGE_CURVE('',#2764,#2779,#2475,.F.);
#3488=EDGE_CURVE('',#2779,#2763,#2476,.F.);
#3489=EDGE_CURVE('',#2775,#2732,#2477,.F.);
#3490=EDGE_CURVE('',#2732,#2776,#2478,.F.);
#3491=EDGE_CURVE('',#2780,#2761,#2479,.F.);
#3492=EDGE_CURVE('',#2762,#2780,#2480,.F.);
#3493=EDGE_CURVE('',#2780,#2779,#1765,.T.);
#3494=EDGE_CURVE('',#2752,#2780,#258,.T.);
#3495=EDGE_CURVE('',#2779,#2753,#259,.T.);
#3496=EDGE_CURVE('',#2781,#2782,#2481,.F.);
#3497=EDGE_CURVE('',#2783,#2781,#2482,.F.);
#3498=EDGE_CURVE('',#2782,#2783,#2483,.F.);
#3499=EDGE_CURVE('',#2784,#2785,#2484,.F.);
#3500=EDGE_CURVE('',#2786,#2784,#2485,.F.);
#3501=EDGE_CURVE('',#2785,#2786,#2486,.F.);
#3502=EDGE_CURVE('',#2787,#2788,#2487,.F.);
#3503=EDGE_CURVE('',#2789,#2787,#2488,.F.);
#3504=EDGE_CURVE('',#2788,#2789,#2489,.F.);
#3505=EDGE_CURVE('',#2782,#2789,#1766,.T.);
#3506=EDGE_CURVE('',#2787,#2781,#1767,.T.);
#3507=EDGE_CURVE('',#2744,#2788,#260,.T.);
#3508=EDGE_CURVE('',#2789,#2745,#261,.T.);
#3509=EDGE_CURVE('',#2790,#2791,#2490,.F.);
#3510=EDGE_CURVE('',#2792,#2790,#2491,.F.);
#3511=EDGE_CURVE('',#2791,#2792,#2492,.F.);
#3512=EDGE_CURVE('',#2790,#2786,#1768,.T.);
#3513=EDGE_CURVE('',#2784,#2792,#1769,.T.);
#3514=EDGE_CURVE('',#2788,#2791,#262,.T.);
#3515=EDGE_CURVE('',#2792,#2787,#263,.T.);
#3516=EDGE_CURVE('',#2742,#2790,#264,.T.);
#3517=EDGE_CURVE('',#2791,#2743,#265,.T.);
#3518=EDGE_CURVE('',#2740,#2785,#266,.T.);
#3519=EDGE_CURVE('',#2786,#2741,#267,.T.);
#3520=EDGE_CURVE('',#2785,#2783,#268,.T.);
#3521=EDGE_CURVE('',#2781,#2784,#269,.T.);
#3522=EDGE_CURVE('',#2738,#2782,#270,.T.);
#3523=EDGE_CURVE('',#2783,#2739,#271,.T.);
#4334=ORIENTED_EDGE('',*,*,#3290,.F.);
#4335=ORIENTED_EDGE('',*,*,#3291,.T.);
#4336=ORIENTED_EDGE('',*,*,#3292,.F.);
#4337=ORIENTED_EDGE('',*,*,#3293,.T.);
#4338=ORIENTED_EDGE('',*,*,#3294,.F.);
#4339=ORIENTED_EDGE('',*,*,#3295,.T.);
#4340=ORIENTED_EDGE('',*,*,#3296,.F.);
#4341=ORIENTED_EDGE('',*,*,#3297,.T.);
#4342=ORIENTED_EDGE('',*,*,#3292,.T.);
#4343=ORIENTED_EDGE('',*,*,#3298,.F.);
#4344=ORIENTED_EDGE('',*,*,#3299,.T.);
#4345=ORIENTED_EDGE('',*,*,#3300,.F.);
#4346=ORIENTED_EDGE('',*,*,#3301,.T.);
#4347=ORIENTED_EDGE('',*,*,#3302,.F.);
#4348=ORIENTED_EDGE('',*,*,#3296,.T.);
#4349=ORIENTED_EDGE('',*,*,#3303,.F.);
#4350=ORIENTED_EDGE('',*,*,#3304,.T.);
#4351=ORIENTED_EDGE('',*,*,#3305,.F.);
#4352=ORIENTED_EDGE('',*,*,#3306,.T.);
#4353=ORIENTED_EDGE('',*,*,#3307,.F.);
#4354=ORIENTED_EDGE('',*,*,#3308,.T.);
#4355=ORIENTED_EDGE('',*,*,#3309,.T.);
#4356=ORIENTED_EDGE('',*,*,#3303,.T.);
#4357=ORIENTED_EDGE('',*,*,#3297,.F.);
#4358=ORIENTED_EDGE('',*,*,#3307,.T.);
#4359=ORIENTED_EDGE('',*,*,#3310,.T.);
#4360=ORIENTED_EDGE('',*,*,#3311,.T.);
#4361=ORIENTED_EDGE('',*,*,#3291,.F.);
#4362=ORIENTED_EDGE('',*,*,#3312,.T.);
#4363=ORIENTED_EDGE('',*,*,#3313,.T.);
#4364=ORIENTED_EDGE('',*,*,#3314,.T.);
#4365=ORIENTED_EDGE('',*,*,#3315,.F.);
#4366=ORIENTED_EDGE('',*,*,#3316,.T.);
#4367=ORIENTED_EDGE('',*,*,#3312,.F.);
#4368=ORIENTED_EDGE('',*,*,#3316,.F.);
#4369=ORIENTED_EDGE('',*,*,#3317,.F.);
#4370=ORIENTED_EDGE('',*,*,#3318,.T.);
#4371=ORIENTED_EDGE('',*,*,#3319,.F.);
#4372=ORIENTED_EDGE('',*,*,#3318,.F.);
#4373=ORIENTED_EDGE('',*,*,#3320,.F.);
#4374=ORIENTED_EDGE('',*,*,#3321,.T.);
#4375=ORIENTED_EDGE('',*,*,#3322,.F.);
#4376=ORIENTED_EDGE('',*,*,#3321,.F.);
#4377=ORIENTED_EDGE('',*,*,#3323,.F.);
#4378=ORIENTED_EDGE('',*,*,#3324,.T.);
#4379=ORIENTED_EDGE('',*,*,#3313,.F.);
#4380=ORIENTED_EDGE('',*,*,#3324,.F.);
#4381=ORIENTED_EDGE('',*,*,#3325,.F.);
#4382=ORIENTED_EDGE('',*,*,#3326,.T.);
#4383=ORIENTED_EDGE('',*,*,#3327,.T.);
#4384=ORIENTED_EDGE('',*,*,#3326,.F.);
#4385=ORIENTED_EDGE('',*,*,#3327,.F.);
#4386=ORIENTED_EDGE('',*,*,#3328,.F.);
#4387=ORIENTED_EDGE('',*,*,#3329,.F.);
#4388=ORIENTED_EDGE('',*,*,#3330,.T.);
#4389=ORIENTED_EDGE('',*,*,#3331,.T.);
#4390=ORIENTED_EDGE('',*,*,#3330,.F.);
#4391=ORIENTED_EDGE('',*,*,#3331,.F.);
#4392=ORIENTED_EDGE('',*,*,#3332,.F.);
#4393=ORIENTED_EDGE('',*,*,#3328,.T.);
#4394=ORIENTED_EDGE('',*,*,#3333,.T.);
#4395=ORIENTED_EDGE('',*,*,#3334,.F.);
#4396=ORIENTED_EDGE('',*,*,#3333,.F.);
#4397=ORIENTED_EDGE('',*,*,#3332,.T.);
#4398=ORIENTED_EDGE('',*,*,#3335,.T.);
#4399=ORIENTED_EDGE('',*,*,#3336,.F.);
#4400=ORIENTED_EDGE('',*,*,#3335,.F.);
#4401=ORIENTED_EDGE('',*,*,#3337,.F.);
#4402=ORIENTED_EDGE('',*,*,#3338,.F.);
#4403=ORIENTED_EDGE('',*,*,#3339,.F.);
#4404=ORIENTED_EDGE('',*,*,#3340,.T.);
#4405=ORIENTED_EDGE('',*,*,#3341,.F.);
#4406=ORIENTED_EDGE('',*,*,#3342,.T.);
#4407=ORIENTED_EDGE('',*,*,#3343,.F.);
#4408=ORIENTED_EDGE('',*,*,#3344,.F.);
#4409=ORIENTED_EDGE('',*,*,#3345,.F.);
#4410=ORIENTED_EDGE('',*,*,#3346,.T.);
#4411=ORIENTED_EDGE('',*,*,#3347,.F.);
#4412=ORIENTED_EDGE('',*,*,#3348,.F.);
#4413=ORIENTED_EDGE('',*,*,#3349,.F.);
#4414=ORIENTED_EDGE('',*,*,#3350,.T.);
#4415=ORIENTED_EDGE('',*,*,#3351,.F.);
#4416=ORIENTED_EDGE('',*,*,#3352,.F.);
#4417=ORIENTED_EDGE('',*,*,#3353,.F.);
#4418=ORIENTED_EDGE('',*,*,#3354,.T.);
#4419=ORIENTED_EDGE('',*,*,#3355,.F.);
#4420=ORIENTED_EDGE('',*,*,#3356,.F.);
#4421=ORIENTED_EDGE('',*,*,#3357,.F.);
#4422=ORIENTED_EDGE('',*,*,#3358,.F.);
#4423=ORIENTED_EDGE('',*,*,#3359,.F.);
#4424=ORIENTED_EDGE('',*,*,#3360,.T.);
#4425=ORIENTED_EDGE('',*,*,#3361,.F.);
#4426=ORIENTED_EDGE('',*,*,#3362,.F.);
#4427=ORIENTED_EDGE('',*,*,#3363,.F.);
#4428=ORIENTED_EDGE('',*,*,#3364,.T.);
#4429=ORIENTED_EDGE('',*,*,#3365,.F.);
#4430=ORIENTED_EDGE('',*,*,#3334,.T.);
#4431=ORIENTED_EDGE('',*,*,#3366,.F.);
#4432=ORIENTED_EDGE('',*,*,#3336,.T.);
#4433=ORIENTED_EDGE('',*,*,#3367,.F.);
#4434=ORIENTED_EDGE('',*,*,#3340,.F.);
#4435=ORIENTED_EDGE('',*,*,#3368,.F.);
#4436=ORIENTED_EDGE('',*,*,#3354,.F.);
#4437=ORIENTED_EDGE('',*,*,#3369,.F.);
#4438=ORIENTED_EDGE('',*,*,#3360,.F.);
#4439=ORIENTED_EDGE('',*,*,#3370,.F.);
#4440=ORIENTED_EDGE('',*,*,#3342,.F.);
#4441=ORIENTED_EDGE('',*,*,#3371,.F.);
#4442=ORIENTED_EDGE('',*,*,#3364,.F.);
#4443=ORIENTED_EDGE('',*,*,#3372,.F.);
#4444=ORIENTED_EDGE('',*,*,#3346,.F.);
#4445=ORIENTED_EDGE('',*,*,#3373,.F.);
#4446=ORIENTED_EDGE('',*,*,#3374,.F.);
#4447=ORIENTED_EDGE('',*,*,#3375,.F.);
#4448=ORIENTED_EDGE('',*,*,#3350,.F.);
#4449=ORIENTED_EDGE('',*,*,#3376,.F.);
#4450=ORIENTED_EDGE('',*,*,#3377,.F.);
#4451=ORIENTED_EDGE('',*,*,#3378,.F.);
#4452=ORIENTED_EDGE('',*,*,#3374,.T.);
#4453=ORIENTED_EDGE('',*,*,#3379,.T.);
#4454=ORIENTED_EDGE('',*,*,#3380,.F.);
#4455=ORIENTED_EDGE('',*,*,#3381,.F.);
#4456=ORIENTED_EDGE('',*,*,#3310,.F.);
#4457=ORIENTED_EDGE('',*,*,#3306,.F.);
#4458=ORIENTED_EDGE('',*,*,#3382,.F.);
#4459=ORIENTED_EDGE('',*,*,#3351,.T.);
#4460=ORIENTED_EDGE('',*,*,#3375,.T.);
#4461=ORIENTED_EDGE('',*,*,#3378,.T.);
#4462=ORIENTED_EDGE('',*,*,#3383,.T.);
#4463=ORIENTED_EDGE('',*,*,#3384,.F.);
#4464=ORIENTED_EDGE('',*,*,#3304,.F.);
#4465=ORIENTED_EDGE('',*,*,#3309,.F.);
#4466=ORIENTED_EDGE('',*,*,#3385,.F.);
#4467=ORIENTED_EDGE('',*,*,#3386,.F.);
#4468=ORIENTED_EDGE('',*,*,#3387,.T.);
#4469=ORIENTED_EDGE('',*,*,#3347,.T.);
#4470=ORIENTED_EDGE('',*,*,#3372,.T.);
#4471=ORIENTED_EDGE('',*,*,#3363,.T.);
#4472=ORIENTED_EDGE('',*,*,#3388,.T.);
#4473=ORIENTED_EDGE('',*,*,#3389,.F.);
#4474=ORIENTED_EDGE('',*,*,#3390,.F.);
#4475=ORIENTED_EDGE('',*,*,#3391,.F.);
#4476=ORIENTED_EDGE('',*,*,#3392,.F.);
#4477=ORIENTED_EDGE('',*,*,#3393,.F.);
#4478=ORIENTED_EDGE('',*,*,#3394,.T.);
#4479=ORIENTED_EDGE('',*,*,#3343,.T.);
#4480=ORIENTED_EDGE('',*,*,#3370,.T.);
#4481=ORIENTED_EDGE('',*,*,#3359,.T.);
#4482=ORIENTED_EDGE('',*,*,#3395,.T.);
#4483=ORIENTED_EDGE('',*,*,#3396,.F.);
#4484=ORIENTED_EDGE('',*,*,#3299,.F.);
#4485=ORIENTED_EDGE('',*,*,#3397,.F.);
#4486=ORIENTED_EDGE('',*,*,#3398,.F.);
#4487=ORIENTED_EDGE('',*,*,#3399,.F.);
#4488=ORIENTED_EDGE('',*,*,#3400,.T.);
#4489=ORIENTED_EDGE('',*,*,#3337,.T.);
#4490=ORIENTED_EDGE('',*,*,#3367,.T.);
#4491=ORIENTED_EDGE('',*,*,#3353,.T.);
#4492=ORIENTED_EDGE('',*,*,#3401,.F.);
#4493=ORIENTED_EDGE('',*,*,#3402,.T.);
#4494=ORIENTED_EDGE('',*,*,#3403,.T.);
#4495=ORIENTED_EDGE('',*,*,#3404,.T.);
#4496=ORIENTED_EDGE('',*,*,#3405,.F.);
#4497=ORIENTED_EDGE('',*,*,#3352,.T.);
#4498=ORIENTED_EDGE('',*,*,#3387,.F.);
#4499=ORIENTED_EDGE('',*,*,#3406,.T.);
#4500=ORIENTED_EDGE('',*,*,#3379,.F.);
#4501=ORIENTED_EDGE('',*,*,#3407,.T.);
#4502=ORIENTED_EDGE('',*,*,#3383,.F.);
#4503=ORIENTED_EDGE('',*,*,#3377,.T.);
#4504=ORIENTED_EDGE('',*,*,#3408,.F.);
#4505=ORIENTED_EDGE('',*,*,#3409,.T.);
#4506=ORIENTED_EDGE('',*,*,#3388,.F.);
#4507=ORIENTED_EDGE('',*,*,#3362,.T.);
#4508=ORIENTED_EDGE('',*,*,#3410,.F.);
#4509=ORIENTED_EDGE('',*,*,#3411,.T.);
#4510=ORIENTED_EDGE('',*,*,#3395,.F.);
#4511=ORIENTED_EDGE('',*,*,#3358,.T.);
#4512=ORIENTED_EDGE('',*,*,#3412,.F.);
#4513=ORIENTED_EDGE('',*,*,#3413,.T.);
#4514=ORIENTED_EDGE('',*,*,#3414,.T.);
#4515=ORIENTED_EDGE('',*,*,#3401,.T.);
#4516=ORIENTED_EDGE('',*,*,#3356,.T.);
#4517=ORIENTED_EDGE('',*,*,#3415,.T.);
#4518=ORIENTED_EDGE('',*,*,#3416,.F.);
#4519=ORIENTED_EDGE('',*,*,#3417,.T.);
#4520=ORIENTED_EDGE('',*,*,#3418,.F.);
#4521=ORIENTED_EDGE('',*,*,#3419,.T.);
#4522=ORIENTED_EDGE('',*,*,#3420,.F.);
#4523=ORIENTED_EDGE('',*,*,#3421,.T.);
#4524=ORIENTED_EDGE('',*,*,#3422,.F.);
#4525=ORIENTED_EDGE('',*,*,#3423,.T.);
#4526=ORIENTED_EDGE('',*,*,#3338,.T.);
#4527=ORIENTED_EDGE('',*,*,#3405,.T.);
#4528=ORIENTED_EDGE('',*,*,#3424,.T.);
#4529=ORIENTED_EDGE('',*,*,#3425,.T.);
#4530=ORIENTED_EDGE('',*,*,#3426,.F.);
#4531=ORIENTED_EDGE('',*,*,#3344,.T.);
#4532=ORIENTED_EDGE('',*,*,#3400,.F.);
#4533=ORIENTED_EDGE('',*,*,#3427,.T.);
#4534=ORIENTED_EDGE('',*,*,#3428,.F.);
#4535=ORIENTED_EDGE('',*,*,#3348,.T.);
#4536=ORIENTED_EDGE('',*,*,#3394,.F.);
#4537=ORIENTED_EDGE('',*,*,#3429,.T.);
#4538=ORIENTED_EDGE('',*,*,#3430,.F.);
#4539=ORIENTED_EDGE('',*,*,#3431,.T.);
#4540=ORIENTED_EDGE('',*,*,#3432,.T.);
#4541=ORIENTED_EDGE('',*,*,#3433,.T.);
#4542=ORIENTED_EDGE('',*,*,#3434,.T.);
#4543=ORIENTED_EDGE('',*,*,#3435,.T.);
#4544=ORIENTED_EDGE('',*,*,#3436,.F.);
#4545=ORIENTED_EDGE('',*,*,#3314,.F.);
#4546=ORIENTED_EDGE('',*,*,#3437,.T.);
#4547=ORIENTED_EDGE('',*,*,#3366,.T.);
#4548=ORIENTED_EDGE('',*,*,#3437,.F.);
#4549=ORIENTED_EDGE('',*,*,#3438,.F.);
#4550=ORIENTED_EDGE('',*,*,#3439,.T.);
#4551=ORIENTED_EDGE('',*,*,#3365,.T.);
#4552=ORIENTED_EDGE('',*,*,#3439,.F.);
#4553=ORIENTED_EDGE('',*,*,#3440,.F.);
#4554=ORIENTED_EDGE('',*,*,#3436,.T.);
#4555=ORIENTED_EDGE('',*,*,#3441,.F.);
#4556=ORIENTED_EDGE('',*,*,#3442,.F.);
#4557=ORIENTED_EDGE('',*,*,#3443,.F.);
#4558=ORIENTED_EDGE('',*,*,#3444,.F.);
#4559=ORIENTED_EDGE('',*,*,#3380,.T.);
#4560=ORIENTED_EDGE('',*,*,#3406,.F.);
#4561=ORIENTED_EDGE('',*,*,#3386,.T.);
#4562=ORIENTED_EDGE('',*,*,#3445,.T.);
#4563=ORIENTED_EDGE('',*,*,#3440,.T.);
#4564=ORIENTED_EDGE('',*,*,#3446,.T.);
#4565=ORIENTED_EDGE('',*,*,#3447,.T.);
#4566=ORIENTED_EDGE('',*,*,#3431,.F.);
#4567=ORIENTED_EDGE('',*,*,#3290,.T.);
#4568=ORIENTED_EDGE('',*,*,#3311,.F.);
#4569=ORIENTED_EDGE('',*,*,#3381,.T.);
#4570=ORIENTED_EDGE('',*,*,#3445,.F.);
#4571=ORIENTED_EDGE('',*,*,#3385,.T.);
#4572=ORIENTED_EDGE('',*,*,#3308,.F.);
#4573=ORIENTED_EDGE('',*,*,#3444,.T.);
#4574=ORIENTED_EDGE('',*,*,#3448,.F.);
#4575=ORIENTED_EDGE('',*,*,#3449,.F.);
#4576=ORIENTED_EDGE('',*,*,#3446,.F.);
#4577=ORIENTED_EDGE('',*,*,#3443,.T.);
#4578=ORIENTED_EDGE('',*,*,#3450,.T.);
#4579=ORIENTED_EDGE('',*,*,#3451,.T.);
#4580=ORIENTED_EDGE('',*,*,#3448,.T.);
#4581=ORIENTED_EDGE('',*,*,#3382,.T.);
#4582=ORIENTED_EDGE('',*,*,#3305,.T.);
#4583=ORIENTED_EDGE('',*,*,#3384,.T.);
#4584=ORIENTED_EDGE('',*,*,#3407,.F.);
#4585=ORIENTED_EDGE('',*,*,#3441,.T.);
#4586=ORIENTED_EDGE('',*,*,#3435,.F.);
#4587=ORIENTED_EDGE('',*,*,#3452,.T.);
#4588=ORIENTED_EDGE('',*,*,#3453,.T.);
#4589=ORIENTED_EDGE('',*,*,#3349,.T.);
#4590=ORIENTED_EDGE('',*,*,#3430,.T.);
#4591=ORIENTED_EDGE('',*,*,#3454,.F.);
#4592=ORIENTED_EDGE('',*,*,#3455,.F.);
#4593=ORIENTED_EDGE('',*,*,#3456,.F.);
#4594=ORIENTED_EDGE('',*,*,#3457,.F.);
#4595=ORIENTED_EDGE('',*,*,#3458,.F.);
#4596=ORIENTED_EDGE('',*,*,#3408,.T.);
#4597=ORIENTED_EDGE('',*,*,#3376,.T.);
#4598=ORIENTED_EDGE('',*,*,#3373,.T.);
#4599=ORIENTED_EDGE('',*,*,#3454,.T.);
#4600=ORIENTED_EDGE('',*,*,#3429,.F.);
#4601=ORIENTED_EDGE('',*,*,#3393,.T.);
#4602=ORIENTED_EDGE('',*,*,#3459,.T.);
#4603=ORIENTED_EDGE('',*,*,#3455,.T.);
#4604=ORIENTED_EDGE('',*,*,#3459,.F.);
#4605=ORIENTED_EDGE('',*,*,#3392,.T.);
#4606=ORIENTED_EDGE('',*,*,#3460,.F.);
#4607=ORIENTED_EDGE('',*,*,#3456,.T.);
#4608=ORIENTED_EDGE('',*,*,#3460,.T.);
#4609=ORIENTED_EDGE('',*,*,#3391,.T.);
#4610=ORIENTED_EDGE('',*,*,#3461,.T.);
#4611=ORIENTED_EDGE('',*,*,#3457,.T.);
#4612=ORIENTED_EDGE('',*,*,#3461,.F.);
#4613=ORIENTED_EDGE('',*,*,#3390,.T.);
#4614=ORIENTED_EDGE('',*,*,#3462,.F.);
#4615=ORIENTED_EDGE('',*,*,#3458,.T.);
#4616=ORIENTED_EDGE('',*,*,#3462,.T.);
#4617=ORIENTED_EDGE('',*,*,#3389,.T.);
#4618=ORIENTED_EDGE('',*,*,#3409,.F.);
#4619=ORIENTED_EDGE('',*,*,#3345,.T.);
#4620=ORIENTED_EDGE('',*,*,#3428,.T.);
#4621=ORIENTED_EDGE('',*,*,#3463,.F.);
#4622=ORIENTED_EDGE('',*,*,#3464,.F.);
#4623=ORIENTED_EDGE('',*,*,#3465,.F.);
#4624=ORIENTED_EDGE('',*,*,#3301,.F.);
#4625=ORIENTED_EDGE('',*,*,#3466,.F.);
#4626=ORIENTED_EDGE('',*,*,#3410,.T.);
#4627=ORIENTED_EDGE('',*,*,#3361,.T.);
#4628=ORIENTED_EDGE('',*,*,#3371,.T.);
#4629=ORIENTED_EDGE('',*,*,#3463,.T.);
#4630=ORIENTED_EDGE('',*,*,#3427,.F.);
#4631=ORIENTED_EDGE('',*,*,#3399,.T.);
#4632=ORIENTED_EDGE('',*,*,#3467,.T.);
#4633=ORIENTED_EDGE('',*,*,#3294,.T.);
#4634=ORIENTED_EDGE('',*,*,#3468,.F.);
#4635=ORIENTED_EDGE('',*,*,#3464,.T.);
#4636=ORIENTED_EDGE('',*,*,#3467,.F.);
#4637=ORIENTED_EDGE('',*,*,#3398,.T.);
#4638=ORIENTED_EDGE('',*,*,#3469,.F.);
#4639=ORIENTED_EDGE('',*,*,#3302,.T.);
#4640=ORIENTED_EDGE('',*,*,#3465,.T.);
#4641=ORIENTED_EDGE('',*,*,#3468,.T.);
#4642=ORIENTED_EDGE('',*,*,#3295,.F.);
#4643=ORIENTED_EDGE('',*,*,#3469,.T.);
#4644=ORIENTED_EDGE('',*,*,#3397,.T.);
#4645=ORIENTED_EDGE('',*,*,#3298,.T.);
#4646=ORIENTED_EDGE('',*,*,#3293,.F.);
#4647=ORIENTED_EDGE('',*,*,#3322,.T.);
#4648=ORIENTED_EDGE('',*,*,#3319,.T.);
#4649=ORIENTED_EDGE('',*,*,#3438,.T.);
#4650=ORIENTED_EDGE('',*,*,#3466,.T.);
#4651=ORIENTED_EDGE('',*,*,#3300,.T.);
#4652=ORIENTED_EDGE('',*,*,#3396,.T.);
#4653=ORIENTED_EDGE('',*,*,#3411,.F.);
#4654=ORIENTED_EDGE('',*,*,#3341,.T.);
#4655=ORIENTED_EDGE('',*,*,#3426,.T.);
#4656=ORIENTED_EDGE('',*,*,#3470,.F.);
#4657=ORIENTED_EDGE('',*,*,#3471,.F.);
#4658=ORIENTED_EDGE('',*,*,#3472,.F.);
#4659=ORIENTED_EDGE('',*,*,#3473,.F.);
#4660=ORIENTED_EDGE('',*,*,#3474,.F.);
#4661=ORIENTED_EDGE('',*,*,#3412,.T.);
#4662=ORIENTED_EDGE('',*,*,#3357,.T.);
#4663=ORIENTED_EDGE('',*,*,#3369,.T.);
#4664=ORIENTED_EDGE('',*,*,#3470,.T.);
#4665=ORIENTED_EDGE('',*,*,#3425,.F.);
#4666=ORIENTED_EDGE('',*,*,#3475,.T.);
#4667=ORIENTED_EDGE('',*,*,#3476,.T.);
#4668=ORIENTED_EDGE('',*,*,#3471,.T.);
#4669=ORIENTED_EDGE('',*,*,#3476,.F.);
#4670=ORIENTED_EDGE('',*,*,#3477,.F.);
#4671=ORIENTED_EDGE('',*,*,#3478,.F.);
#4672=ORIENTED_EDGE('',*,*,#3472,.T.);
#4673=ORIENTED_EDGE('',*,*,#3478,.T.);
#4674=ORIENTED_EDGE('',*,*,#3479,.T.);
#4675=ORIENTED_EDGE('',*,*,#3480,.T.);
#4676=ORIENTED_EDGE('',*,*,#3474,.T.);
#4677=ORIENTED_EDGE('',*,*,#3481,.T.);
#4678=ORIENTED_EDGE('',*,*,#3482,.T.);
#4679=ORIENTED_EDGE('',*,*,#3413,.F.);
#4680=ORIENTED_EDGE('',*,*,#3473,.T.);
#4681=ORIENTED_EDGE('',*,*,#3480,.F.);
#4682=ORIENTED_EDGE('',*,*,#3483,.F.);
#4683=ORIENTED_EDGE('',*,*,#3481,.F.);
#4684=ORIENTED_EDGE('',*,*,#3484,.T.);
#4685=ORIENTED_EDGE('',*,*,#3485,.T.);
#4686=ORIENTED_EDGE('',*,*,#3483,.T.);
#4687=ORIENTED_EDGE('',*,*,#3486,.T.);
#4688=ORIENTED_EDGE('',*,*,#3487,.T.);
#4689=ORIENTED_EDGE('',*,*,#3488,.T.);
#4690=ORIENTED_EDGE('',*,*,#3477,.T.);
#4691=ORIENTED_EDGE('',*,*,#3489,.T.);
#4692=ORIENTED_EDGE('',*,*,#3490,.T.);
#4693=ORIENTED_EDGE('',*,*,#3484,.F.);
#4694=ORIENTED_EDGE('',*,*,#3479,.F.);
#4695=ORIENTED_EDGE('',*,*,#3490,.F.);
#4696=ORIENTED_EDGE('',*,*,#3403,.F.);
#4697=ORIENTED_EDGE('',*,*,#3424,.F.);
#4698=ORIENTED_EDGE('',*,*,#3404,.F.);
#4699=ORIENTED_EDGE('',*,*,#3489,.F.);
#4700=ORIENTED_EDGE('',*,*,#3475,.F.);
#4701=ORIENTED_EDGE('',*,*,#3491,.T.);
#4702=ORIENTED_EDGE('',*,*,#3449,.T.);
#4703=ORIENTED_EDGE('',*,*,#3492,.T.);
#4704=ORIENTED_EDGE('',*,*,#3492,.F.);
#4705=ORIENTED_EDGE('',*,*,#3451,.F.);
#4706=ORIENTED_EDGE('',*,*,#3488,.F.);
#4707=ORIENTED_EDGE('',*,*,#3493,.F.);
#4708=ORIENTED_EDGE('',*,*,#3432,.F.);
#4709=ORIENTED_EDGE('',*,*,#3447,.F.);
#4710=ORIENTED_EDGE('',*,*,#3491,.F.);
#4711=ORIENTED_EDGE('',*,*,#3494,.F.);
#4712=ORIENTED_EDGE('',*,*,#3434,.F.);
#4713=ORIENTED_EDGE('',*,*,#3495,.F.);
#4714=ORIENTED_EDGE('',*,*,#3487,.F.);
#4715=ORIENTED_EDGE('',*,*,#3452,.F.);
#4716=ORIENTED_EDGE('',*,*,#3442,.T.);
#4717=ORIENTED_EDGE('',*,*,#3453,.F.);
#4718=ORIENTED_EDGE('',*,*,#3486,.F.);
#4719=ORIENTED_EDGE('',*,*,#3450,.F.);
#4720=ORIENTED_EDGE('',*,*,#3414,.F.);
#4721=ORIENTED_EDGE('',*,*,#3482,.F.);
#4722=ORIENTED_EDGE('',*,*,#3485,.F.);
#4723=ORIENTED_EDGE('',*,*,#3402,.F.);
#4724=ORIENTED_EDGE('',*,*,#3494,.T.);
#4725=ORIENTED_EDGE('',*,*,#3493,.T.);
#4726=ORIENTED_EDGE('',*,*,#3495,.T.);
#4727=ORIENTED_EDGE('',*,*,#3433,.F.);
#4728=ORIENTED_EDGE('',*,*,#3496,.F.);
#4729=ORIENTED_EDGE('',*,*,#3497,.F.);
#4730=ORIENTED_EDGE('',*,*,#3498,.F.);
#4731=ORIENTED_EDGE('',*,*,#3499,.F.);
#4732=ORIENTED_EDGE('',*,*,#3500,.F.);
#4733=ORIENTED_EDGE('',*,*,#3501,.F.);
#4734=ORIENTED_EDGE('',*,*,#3502,.F.);
#4735=ORIENTED_EDGE('',*,*,#3503,.F.);
#4736=ORIENTED_EDGE('',*,*,#3504,.F.);
#4737=ORIENTED_EDGE('',*,*,#3496,.T.);
#4738=ORIENTED_EDGE('',*,*,#3505,.T.);
#4739=ORIENTED_EDGE('',*,*,#3503,.T.);
#4740=ORIENTED_EDGE('',*,*,#3506,.T.);
#4741=ORIENTED_EDGE('',*,*,#3422,.T.);
#4742=ORIENTED_EDGE('',*,*,#3507,.T.);
#4743=ORIENTED_EDGE('',*,*,#3504,.T.);
#4744=ORIENTED_EDGE('',*,*,#3508,.T.);
#4745=ORIENTED_EDGE('',*,*,#3509,.F.);
#4746=ORIENTED_EDGE('',*,*,#3510,.F.);
#4747=ORIENTED_EDGE('',*,*,#3511,.F.);
#4748=ORIENTED_EDGE('',*,*,#3510,.T.);
#4749=ORIENTED_EDGE('',*,*,#3512,.T.);
#4750=ORIENTED_EDGE('',*,*,#3500,.T.);
#4751=ORIENTED_EDGE('',*,*,#3513,.T.);
#4752=ORIENTED_EDGE('',*,*,#3502,.T.);
#4753=ORIENTED_EDGE('',*,*,#3514,.T.);
#4754=ORIENTED_EDGE('',*,*,#3511,.T.);
#4755=ORIENTED_EDGE('',*,*,#3515,.T.);
#4756=ORIENTED_EDGE('',*,*,#3420,.T.);
#4757=ORIENTED_EDGE('',*,*,#3516,.T.);
#4758=ORIENTED_EDGE('',*,*,#3509,.T.);
#4759=ORIENTED_EDGE('',*,*,#3517,.T.);
#4760=ORIENTED_EDGE('',*,*,#3418,.T.);
#4761=ORIENTED_EDGE('',*,*,#3518,.T.);
#4762=ORIENTED_EDGE('',*,*,#3501,.T.);
#4763=ORIENTED_EDGE('',*,*,#3519,.T.);
#4764=ORIENTED_EDGE('',*,*,#3499,.T.);
#4765=ORIENTED_EDGE('',*,*,#3520,.T.);
#4766=ORIENTED_EDGE('',*,*,#3497,.T.);
#4767=ORIENTED_EDGE('',*,*,#3521,.T.);
#4768=ORIENTED_EDGE('',*,*,#3416,.T.);
#4769=ORIENTED_EDGE('',*,*,#3522,.T.);
#4770=ORIENTED_EDGE('',*,*,#3498,.T.);
#4771=ORIENTED_EDGE('',*,*,#3523,.T.);
#4772=ORIENTED_EDGE('',*,*,#3517,.F.);
#4773=ORIENTED_EDGE('',*,*,#3514,.F.);
#4774=ORIENTED_EDGE('',*,*,#3507,.F.);
#4775=ORIENTED_EDGE('',*,*,#3421,.F.);
#4776=ORIENTED_EDGE('',*,*,#3339,.T.);
#4777=ORIENTED_EDGE('',*,*,#3423,.F.);
#4778=ORIENTED_EDGE('',*,*,#3508,.F.);
#4779=ORIENTED_EDGE('',*,*,#3505,.F.);
#4780=ORIENTED_EDGE('',*,*,#3522,.F.);
#4781=ORIENTED_EDGE('',*,*,#3415,.F.);
#4782=ORIENTED_EDGE('',*,*,#3355,.T.);
#4783=ORIENTED_EDGE('',*,*,#3368,.T.);
#4784=ORIENTED_EDGE('',*,*,#3513,.F.);
#4785=ORIENTED_EDGE('',*,*,#3521,.F.);
#4786=ORIENTED_EDGE('',*,*,#3506,.F.);
#4787=ORIENTED_EDGE('',*,*,#3515,.F.);
#4788=ORIENTED_EDGE('',*,*,#3329,.T.);
#4789=ORIENTED_EDGE('',*,*,#3325,.T.);
#4790=ORIENTED_EDGE('',*,*,#3323,.T.);
#4791=ORIENTED_EDGE('',*,*,#3320,.T.);
#4792=ORIENTED_EDGE('',*,*,#3317,.T.);
#4793=ORIENTED_EDGE('',*,*,#3315,.T.);
#4794=ORIENTED_EDGE('',*,*,#3518,.F.);
#4795=ORIENTED_EDGE('',*,*,#3417,.F.);
#4796=ORIENTED_EDGE('',*,*,#3523,.F.);
#4797=ORIENTED_EDGE('',*,*,#3520,.F.);
#4798=ORIENTED_EDGE('',*,*,#3516,.F.);
#4799=ORIENTED_EDGE('',*,*,#3419,.F.);
#4800=ORIENTED_EDGE('',*,*,#3519,.F.);
#4801=ORIENTED_EDGE('',*,*,#3512,.F.);
#6045=CYLINDRICAL_SURFACE('',#6723,0.25);
#6046=CYLINDRICAL_SURFACE('',#6725,0.25);
#6047=CYLINDRICAL_SURFACE('',#6727,0.25);
#6048=CYLINDRICAL_SURFACE('',#6729,0.25);
#6049=CYLINDRICAL_SURFACE('',#6735,0.15);
#6050=CYLINDRICAL_SURFACE('',#6737,0.15);
#6051=CYLINDRICAL_SURFACE('',#6740,0.15);
#6052=CYLINDRICAL_SURFACE('',#6743,0.15);
#6053=CYLINDRICAL_SURFACE('',#6745,0.3);
#6054=CYLINDRICAL_SURFACE('',#6750,0.3);
#6055=CYLINDRICAL_SURFACE('',#6755,0.17);
#6056=CYLINDRICAL_SURFACE('',#6757,0.17);
#6057=CYLINDRICAL_SURFACE('',#6781,0.4);
#6058=CYLINDRICAL_SURFACE('',#6782,0.4);
#6059=CYLINDRICAL_SURFACE('',#6805,0.1);
#6060=CYLINDRICAL_SURFACE('',#6809,0.1);
#6061=CYLINDRICAL_SURFACE('',#6823,0.3);
#6062=CYLINDRICAL_SURFACE('',#6828,0.3);
#6210=ADVANCED_FACE('',(#838),#6045,.F.);
#6211=ADVANCED_FACE('',(#839),#6046,.F.);
#6212=ADVANCED_FACE('',(#840),#6047,.F.);
#6213=ADVANCED_FACE('',(#841),#6048,.F.);
#6214=ADVANCED_FACE('',(#842),#92,.T.);
#6215=ADVANCED_FACE('',(#843),#93,.T.);
#6216=ADVANCED_FACE('',(#844,#599,#600,#601),#682,.F.);
#6217=ADVANCED_FACE('',(#845),#6049,.F.);
#6218=ADVANCED_FACE('',(#846),#6050,.F.);
#6219=ADVANCED_FACE('',(#847),#6051,.F.);
#6220=ADVANCED_FACE('',(#848),#6052,.F.);
#6221=ADVANCED_FACE('',(#849),#6053,.F.);
#6222=ADVANCED_FACE('',(#850,#602),#683,.F.);
#6223=ADVANCED_FACE('',(#851),#6054,.F.);
#6224=ADVANCED_FACE('',(#852,#603),#684,.F.);
#6225=ADVANCED_FACE('',(#853),#6055,.F.);
#6226=ADVANCED_FACE('',(#854),#6056,.F.);
#6227=ADVANCED_FACE('',(#855),#685,.F.);
#6228=ADVANCED_FACE('',(#856),#686,.F.);
#6229=ADVANCED_FACE('',(#857),#687,.F.);
#6230=ADVANCED_FACE('',(#858),#688,.F.);
#6231=ADVANCED_FACE('',(#859),#689,.F.);
#6232=ADVANCED_FACE('',(#860),#690,.F.);
#6233=ADVANCED_FACE('',(#861),#691,.F.);
#6234=ADVANCED_FACE('',(#862,#604),#692,.F.);
#6235=ADVANCED_FACE('',(#863,#605),#693,.F.);
#6236=ADVANCED_FACE('',(#864),#694,.F.);
#6237=ADVANCED_FACE('',(#865),#695,.F.);
#6238=ADVANCED_FACE('',(#866),#696,.F.);
#6239=ADVANCED_FACE('',(#867),#697,.F.);
#6240=ADVANCED_FACE('',(#868),#698,.F.);
#6241=ADVANCED_FACE('',(#869),#699,.T.);
#6242=ADVANCED_FACE('',(#870),#700,.T.);
#6243=ADVANCED_FACE('',(#871),#701,.T.);
#6244=ADVANCED_FACE('',(#872),#702,.T.);
#6245=ADVANCED_FACE('',(#873),#703,.T.);
#6246=ADVANCED_FACE('',(#874,#606),#704,.F.);
#6247=ADVANCED_FACE('',(#875),#6057,.T.);
#6248=ADVANCED_FACE('',(#876),#6058,.T.);
#6249=ADVANCED_FACE('',(#877),#705,.T.);
#6250=ADVANCED_FACE('',(#878),#94,.T.);
#6251=ADVANCED_FACE('',(#879),#95,.T.);
#6252=ADVANCED_FACE('',(#880),#96,.T.);
#6253=ADVANCED_FACE('',(#881),#97,.T.);
#6254=ADVANCED_FACE('',(#882),#706,.F.);
#6255=ADVANCED_FACE('',(#883),#98,.T.);
#6256=ADVANCED_FACE('',(#884),#99,.T.);
#6257=ADVANCED_FACE('',(#885),#707,.T.);
#6258=ADVANCED_FACE('',(#886),#100,.T.);
#6259=ADVANCED_FACE('',(#887),#101,.T.);
#6260=ADVANCED_FACE('',(#888),#708,.F.);
#6261=ADVANCED_FACE('',(#889),#102,.T.);
#6262=ADVANCED_FACE('',(#890),#103,.T.);
#6263=ADVANCED_FACE('',(#891),#709,.T.);
#6264=ADVANCED_FACE('',(#892),#104,.T.);
#6265=ADVANCED_FACE('',(#893),#105,.T.);
#6266=ADVANCED_FACE('',(#894,#607,#608,#609),#710,.F.);
#6267=ADVANCED_FACE('',(#895),#106,.T.);
#6268=ADVANCED_FACE('',(#896),#711,.T.);
#6269=ADVANCED_FACE('',(#897),#107,.T.);
#6270=ADVANCED_FACE('',(#898),#108,.T.);
#6271=ADVANCED_FACE('',(#899),#712,.F.);
#6272=ADVANCED_FACE('',(#900),#109,.T.);
#6273=ADVANCED_FACE('',(#901),#110,.T.);
#6274=ADVANCED_FACE('',(#902),#76,.F.);
#6275=ADVANCED_FACE('',(#903),#77,.F.);
#6276=ADVANCED_FACE('',(#904),#78,.F.);
#6277=ADVANCED_FACE('',(#905),#6059,.F.);
#6278=ADVANCED_FACE('',(#906),#111,.T.);
#6279=ADVANCED_FACE('',(#907),#79,.F.);
#6280=ADVANCED_FACE('',(#908),#6060,.F.);
#6281=ADVANCED_FACE('',(#909),#112,.T.);
#6282=ADVANCED_FACE('',(#910),#113,.T.);
#6283=ADVANCED_FACE('',(#911),#114,.T.);
#6284=ADVANCED_FACE('',(#912),#115,.T.);
#6285=ADVANCED_FACE('',(#913),#713,.T.);
#6286=ADVANCED_FACE('',(#914),#80,.T.);
#6287=ADVANCED_FACE('',(#915),#81,.T.);
#6288=ADVANCED_FACE('',(#916),#82,.T.);
#6289=ADVANCED_FACE('',(#917),#6061,.T.);
#6290=ADVANCED_FACE('',(#918),#116,.F.);
#6291=ADVANCED_FACE('',(#919),#83,.T.);
#6292=ADVANCED_FACE('',(#920),#6062,.T.);
#6293=ADVANCED_FACE('',(#921),#117,.F.);
#6294=ADVANCED_FACE('',(#922),#118,.F.);
#6295=ADVANCED_FACE('',(#923),#119,.F.);
#6296=ADVANCED_FACE('',(#924),#120,.F.);
#6297=ADVANCED_FACE('',(#925),#121,.F.);
#6298=ADVANCED_FACE('',(#926),#122,.F.);
#6299=ADVANCED_FACE('',(#927),#714,.F.);
#6300=ADVANCED_FACE('',(#928,#610,#611,#612,#613,#614,#615),#715,.T.);
#6301=ADVANCED_FACE('',(#929),#123,.F.);
#6302=ADVANCED_FACE('',(#930),#716,.F.);
#6547=CLOSED_SHELL('',(#6210,#6211,#6212,#6213,#6214,#6215,#6216,#6217,
#6218,#6219,#6220,#6221,#6222,#6223,#6224,#6225,#6226,#6227,#6228,#6229,
#6230,#6231,#6232,#6233,#6234,#6235,#6236,#6237,#6238,#6239,#6240,#6241,
#6242,#6243,#6244,#6245,#6246,#6247,#6248,#6249,#6250,#6251,#6252,#6253,
#6254,#6255,#6256,#6257,#6258,#6259,#6260,#6261,#6262,#6263,#6264,#6265,
#6266,#6267,#6268,#6269,#6270,#6271,#6272,#6273,#6274,#6275,#6276,#6277,
#6278,#6279,#6280,#6281,#6282,#6283,#6284,#6285,#6286,#6287,#6288,#6289,
#6290,#6291,#6292,#6293,#6294,#6295,#6296,#6297,#6298,#6299,#6300,#6301,
#6302));
#6722=AXIS2_PLACEMENT_3D('',#8711,#7347,#7348);
#6723=AXIS2_PLACEMENT_3D('',#8712,#7349,#7350);
#6724=AXIS2_PLACEMENT_3D('',#8739,#7351,#7352);
#6725=AXIS2_PLACEMENT_3D('',#8740,#7353,#7354);
#6726=AXIS2_PLACEMENT_3D('',#8763,#7355,#7356);
#6727=AXIS2_PLACEMENT_3D('',#8764,#7357,#7358);
#6728=AXIS2_PLACEMENT_3D('',#8787,#7359,#7360);
#6729=AXIS2_PLACEMENT_3D('',#8788,#7361,#7362);
#6730=AXIS2_PLACEMENT_3D('',#8815,#7363,#7364);
#6731=AXIS2_PLACEMENT_3D('',#9000,#7365,#7366);
#6732=AXIS2_PLACEMENT_3D('',#9014,#7369,#7370);
#6733=AXIS2_PLACEMENT_3D('',#9016,#7371,#7372);
#6734=AXIS2_PLACEMENT_3D('',#9018,#7373,#7374);
#6735=AXIS2_PLACEMENT_3D('',#9019,#7375,#7376);
#6736=AXIS2_PLACEMENT_3D('',#9021,#7377,#7378);
#6737=AXIS2_PLACEMENT_3D('',#9023,#7380,#7381);
#6738=AXIS2_PLACEMENT_3D('',#9025,#7382,#7383);
#6739=AXIS2_PLACEMENT_3D('',#9028,#7385,#7386);
#6740=AXIS2_PLACEMENT_3D('',#9029,#7387,#7388);
#6741=AXIS2_PLACEMENT_3D('',#9031,#7389,#7390);
#6742=AXIS2_PLACEMENT_3D('',#9034,#7392,#7393);
#6743=AXIS2_PLACEMENT_3D('',#9035,#7394,#7395);
#6744=AXIS2_PLACEMENT_3D('',#9037,#7396,#7397);
#6745=AXIS2_PLACEMENT_3D('',#9039,#7399,#7400);
#6746=AXIS2_PLACEMENT_3D('',#9041,#7401,#7402);
#6747=AXIS2_PLACEMENT_3D('',#9044,#7404,#7405);
#6748=AXIS2_PLACEMENT_3D('',#9045,#7406,#7407);
#6749=AXIS2_PLACEMENT_3D('',#9047,#7408,#7409);
#6750=AXIS2_PLACEMENT_3D('',#9048,#7410,#7411);
#6751=AXIS2_PLACEMENT_3D('',#9050,#7412,#7413);
#6752=AXIS2_PLACEMENT_3D('',#9053,#7415,#7416);
#6753=AXIS2_PLACEMENT_3D('',#9054,#7417,#7418);
#6754=AXIS2_PLACEMENT_3D('',#9056,#7419,#7420);
#6755=AXIS2_PLACEMENT_3D('',#9057,#7421,#7422);
#6756=AXIS2_PLACEMENT_3D('',#9060,#7424,#7425);
#6757=AXIS2_PLACEMENT_3D('',#9061,#7426,#7427);
#6758=AXIS2_PLACEMENT_3D('',#9064,#7429,#7430);
#6759=AXIS2_PLACEMENT_3D('',#9065,#7431,#7432);
#6760=AXIS2_PLACEMENT_3D('',#9074,#7437,#7438);
#6761=AXIS2_PLACEMENT_3D('',#9083,#7443,#7444);
#6762=AXIS2_PLACEMENT_3D('',#9092,#7449,#7450);
#6763=AXIS2_PLACEMENT_3D('',#9101,#7455,#7456);
#6764=AXIS2_PLACEMENT_3D('',#9110,#7461,#7462);
#6765=AXIS2_PLACEMENT_3D('',#9119,#7467,#7468);
#6766=AXIS2_PLACEMENT_3D('',#9128,#7473,#7474);
#6767=AXIS2_PLACEMENT_3D('',#9130,#7475,#7476);
#6768=AXIS2_PLACEMENT_3D('',#9131,#7477,#7478);
#6769=AXIS2_PLACEMENT_3D('',#9133,#7479,#7480);
#6770=AXIS2_PLACEMENT_3D('',#9134,#7481,#7482);
#6771=AXIS2_PLACEMENT_3D('',#9137,#7485,#7486);
#6772=AXIS2_PLACEMENT_3D('',#9140,#7489,#7490);
#6773=AXIS2_PLACEMENT_3D('',#9143,#7493,#7494);
#6774=AXIS2_PLACEMENT_3D('',#9149,#7498,#7499);
#6775=AXIS2_PLACEMENT_3D('',#9155,#7503,#7504);
#6776=AXIS2_PLACEMENT_3D('',#9200,#7506,#7507);
#6777=AXIS2_PLACEMENT_3D('',#9246,#7510,#7511);
#6778=AXIS2_PLACEMENT_3D('',#9324,#7515,#7516);
#6779=AXIS2_PLACEMENT_3D('',#9372,#7520,#7521);
#6780=AXIS2_PLACEMENT_3D('',#9388,#7525,#7526);
#6781=AXIS2_PLACEMENT_3D('',#9709,#7538,#7539);
#6782=AXIS2_PLACEMENT_3D('',#9711,#7541,#7542);
#6783=AXIS2_PLACEMENT_3D('',#9713,#7543,#7544);
#6784=AXIS2_PLACEMENT_3D('',#9715,#7546,#7547);
#6785=AXIS2_PLACEMENT_3D('',#9879,#7549,#7550);
#6786=AXIS2_PLACEMENT_3D('',#9880,#7551,#7552);
#6787=AXIS2_PLACEMENT_3D('',#9928,#7554,#7555);
#6788=AXIS2_PLACEMENT_3D('',#10046,#7557,#7558);
#6789=AXIS2_PLACEMENT_3D('',#10091,#7559,#7560);
#6790=AXIS2_PLACEMENT_3D('',#10183,#7562,#7563);
#6791=AXIS2_PLACEMENT_3D('',#10200,#7564,#7565);
#6792=AXIS2_PLACEMENT_3D('',#10320,#7567,#7568);
#6793=AXIS2_PLACEMENT_3D('',#10325,#7569,#7570);
#6794=AXIS2_PLACEMENT_3D('',#10377,#7572,#7573);
#6795=AXIS2_PLACEMENT_3D('',#10378,#7574,#7575);
#6796=AXIS2_PLACEMENT_3D('',#10379,#7576,#7577);
#6797=AXIS2_PLACEMENT_3D('',#10380,#7578,#7579);
#6798=AXIS2_PLACEMENT_3D('',#10381,#7580,#7581);
#6799=AXIS2_PLACEMENT_3D('',#10382,#7582,#7583);
#6800=AXIS2_PLACEMENT_3D('',#10384,#7584,#7585);
#6801=AXIS2_PLACEMENT_3D('',#10385,#7586,#7587);
#6802=AXIS2_PLACEMENT_3D('',#10386,#7588,#7589);
#6803=AXIS2_PLACEMENT_3D('',#10387,#7590,#7591);
#6804=AXIS2_PLACEMENT_3D('',#10388,#7592,#7593);
#6805=AXIS2_PLACEMENT_3D('',#10389,#7594,#7595);
#6806=AXIS2_PLACEMENT_3D('',#10410,#7596,#7597);
#6807=AXIS2_PLACEMENT_3D('',#10412,#7598,#7599);
#6808=AXIS2_PLACEMENT_3D('',#10413,#7600,#7601);
#6809=AXIS2_PLACEMENT_3D('',#10414,#7602,#7603);
#6810=AXIS2_PLACEMENT_3D('',#10504,#7605,#7606);
#6811=AXIS2_PLACEMENT_3D('',#10505,#7607,#7608);
#6812=AXIS2_PLACEMENT_3D('',#10508,#7609,#7610);
#6813=AXIS2_PLACEMENT_3D('',#10510,#7611,#7612);
#6814=AXIS2_PLACEMENT_3D('',#10511,#7613,#7614);
#6815=AXIS2_PLACEMENT_3D('',#10512,#7615,#7616);
#6816=AXIS2_PLACEMENT_3D('',#10515,#7617,#7618);
#6817=AXIS2_PLACEMENT_3D('',#10517,#7619,#7620);
#6818=AXIS2_PLACEMENT_3D('',#10518,#7621,#7622);
#6819=AXIS2_PLACEMENT_3D('',#10519,#7623,#7624);
#6820=AXIS2_PLACEMENT_3D('',#10522,#7625,#7626);
#6821=AXIS2_PLACEMENT_3D('',#10524,#7627,#7628);
#6822=AXIS2_PLACEMENT_3D('',#10525,#7629,#7630);
#6823=AXIS2_PLACEMENT_3D('',#10526,#7631,#7632);
#6824=AXIS2_PLACEMENT_3D('',#10557,#7635,#7636);
#6825=AXIS2_PLACEMENT_3D('',#10560,#7637,#7638);
#6826=AXIS2_PLACEMENT_3D('',#10562,#7639,#7640);
#6827=AXIS2_PLACEMENT_3D('',#10563,#7641,#7642);
#6828=AXIS2_PLACEMENT_3D('',#10564,#7643,#7644);
#6829=AXIS2_PLACEMENT_3D('',#10737,#7647,#7648);
#6830=AXIS2_PLACEMENT_3D('',#10738,#7649,#7650);
#6831=AXIS2_PLACEMENT_3D('',#10755,#7651,#7652);
#7347=DIRECTION('axis',(0.,0.,1.));
#7348=DIRECTION('refdir',(1.,0.,0.));
#7349=DIRECTION('center_axis',(0.,0.,-1.));
#7350=DIRECTION('ref_axis',(1.,0.,0.));
#7351=DIRECTION('center_axis',(0.,0.,1.));
#7352=DIRECTION('ref_axis',(1.,0.,0.));
#7353=DIRECTION('center_axis',(0.,0.,-1.));
#7354=DIRECTION('ref_axis',(1.,0.,0.));
#7355=DIRECTION('center_axis',(0.,0.,1.));
#7356=DIRECTION('ref_axis',(1.,0.,0.));
#7357=DIRECTION('center_axis',(0.,0.,-1.));
#7358=DIRECTION('ref_axis',(1.,0.,0.));
#7359=DIRECTION('center_axis',(0.,0.,1.));
#7360=DIRECTION('ref_axis',(1.,0.,0.));
#7361=DIRECTION('center_axis',(0.,0.,-1.));
#7362=DIRECTION('ref_axis',(1.,0.,0.));
#7363=DIRECTION('center_axis',(0.,0.,1.));
#7364=DIRECTION('ref_axis',(1.,0.,0.));
#7365=DIRECTION('center_axis',(4.10828654779316E-33,-1.13946463231163E-19,
1.));
#7366=DIRECTION('ref_axis',(1.,0.,-4.10828654779316E-33));
#7367=DIRECTION('',(0.,1.,1.13946463231163E-19));
#7368=DIRECTION('',(0.,-1.,-1.13946463231163E-19));
#7369=DIRECTION('center_axis',(4.10828654779316E-33,-1.13946463231163E-19,
1.));
#7370=DIRECTION('ref_axis',(1.,0.,0.));
#7371=DIRECTION('center_axis',(4.10828654779316E-33,-1.13946463231163E-19,
1.));
#7372=DIRECTION('ref_axis',(1.,0.,0.));
#7373=DIRECTION('center_axis',(4.10828654779316E-33,-1.13946463231163E-19,
1.));
#7374=DIRECTION('ref_axis',(1.,0.,0.));
#7375=DIRECTION('center_axis',(0.,0.,-1.));
#7376=DIRECTION('ref_axis',(1.,0.,0.));
#7377=DIRECTION('center_axis',(-4.10828654779316E-33,1.13946463231163E-19,
-1.));
#7378=DIRECTION('ref_axis',(1.,0.,0.));
#7379=DIRECTION('',(0.,0.,-1.));
#7380=DIRECTION('center_axis',(0.,0.,-1.));
#7381=DIRECTION('ref_axis',(1.,0.,0.));
#7382=DIRECTION('center_axis',(-4.10828654779316E-33,1.13946463231163E-19,
-1.));
#7383=DIRECTION('ref_axis',(1.,0.,0.));
#7384=DIRECTION('',(0.,0.,-1.));
#7385=DIRECTION('center_axis',(4.10828654779316E-33,-1.13946463231163E-19,
1.));
#7386=DIRECTION('ref_axis',(1.,0.,0.));
#7387=DIRECTION('center_axis',(0.,0.,-1.));
#7388=DIRECTION('ref_axis',(1.,0.,0.));
#7389=DIRECTION('center_axis',(-4.10828654779316E-33,1.13946463231163E-19,
-1.));
#7390=DIRECTION('ref_axis',(1.,0.,0.));
#7391=DIRECTION('',(0.,0.,-1.));
#7392=DIRECTION('center_axis',(4.10828654779316E-33,-1.13946463231163E-19,
1.));
#7393=DIRECTION('ref_axis',(1.,0.,0.));
#7394=DIRECTION('center_axis',(0.,0.,-1.));
#7395=DIRECTION('ref_axis',(1.,0.,0.));
#7396=DIRECTION('center_axis',(-4.10828654779316E-33,1.13946463231163E-19,
-1.));
#7397=DIRECTION('ref_axis',(1.,0.,0.));
#7398=DIRECTION('',(0.,0.,-1.));
#7399=DIRECTION('center_axis',(0.,0.,-1.));
#7400=DIRECTION('ref_axis',(1.,0.,0.));
#7401=DIRECTION('center_axis',(-4.10828654779316E-33,1.13946463231163E-19,
-1.));
#7402=DIRECTION('ref_axis',(1.,0.,0.));
#7403=DIRECTION('',(0.,0.,-1.));
#7404=DIRECTION('center_axis',(0.,0.,-1.));
#7405=DIRECTION('ref_axis',(1.,0.,0.));
#7406=DIRECTION('center_axis',(0.,0.,-1.));
#7407=DIRECTION('ref_axis',(1.,0.,0.));
#7408=DIRECTION('center_axis',(0.,0.,1.));
#7409=DIRECTION('ref_axis',(1.,0.,0.));
#7410=DIRECTION('center_axis',(0.,0.,-1.));
#7411=DIRECTION('ref_axis',(1.,0.,0.));
#7412=DIRECTION('center_axis',(-4.10828654779316E-33,1.13946463231163E-19,
-1.));
#7413=DIRECTION('ref_axis',(1.,0.,0.));
#7414=DIRECTION('',(0.,0.,-1.));
#7415=DIRECTION('center_axis',(0.,0.,-1.));
#7416=DIRECTION('ref_axis',(1.,0.,0.));
#7417=DIRECTION('center_axis',(0.,0.,-1.));
#7418=DIRECTION('ref_axis',(1.,0.,0.));
#7419=DIRECTION('center_axis',(0.,0.,1.));
#7420=DIRECTION('ref_axis',(1.,0.,0.));
#7421=DIRECTION('center_axis',(0.,0.,-1.));
#7422=DIRECTION('ref_axis',(1.,0.,0.));
#7423=DIRECTION('',(0.,0.,-1.));
#7424=DIRECTION('center_axis',(0.,0.,1.));
#7425=DIRECTION('ref_axis',(1.,0.,0.));
#7426=DIRECTION('center_axis',(0.,0.,-1.));
#7427=DIRECTION('ref_axis',(1.,0.,0.));
#7428=DIRECTION('',(0.,0.,-1.));
#7429=DIRECTION('center_axis',(0.,0.,1.));
#7430=DIRECTION('ref_axis',(1.,0.,0.));
#7431=DIRECTION('center_axis',(0.,-1.,0.));
#7432=DIRECTION('ref_axis',(-1.,0.,0.));
#7433=DIRECTION('',(0.0523359562429438,0.,0.998629534754574));
#7434=DIRECTION('',(1.,0.,0.));
#7435=DIRECTION('',(-0.0523359562429438,0.,-0.998629534754574));
#7436=DIRECTION('',(1.,0.,0.));
#7437=DIRECTION('center_axis',(0.,-1.,0.));
#7438=DIRECTION('ref_axis',(-1.,0.,0.));
#7439=DIRECTION('',(0.,0.,-1.));
#7440=DIRECTION('',(1.,0.,0.));
#7441=DIRECTION('',(0.,0.,1.));
#7442=DIRECTION('',(1.,0.,0.));
#7443=DIRECTION('center_axis',(0.,-1.,0.));
#7444=DIRECTION('ref_axis',(-1.,0.,0.));
#7445=DIRECTION('',(0.,0.,-1.));
#7446=DIRECTION('',(1.,0.,0.));
#7447=DIRECTION('',(0.,0.,1.));
#7448=DIRECTION('',(1.,0.,0.));
#7449=DIRECTION('center_axis',(0.,-1.,0.));
#7450=DIRECTION('ref_axis',(-1.,0.,0.));
#7451=DIRECTION('',(0.,0.,-1.));
#7452=DIRECTION('',(1.,0.,0.));
#7453=DIRECTION('',(0.,0.,1.));
#7454=DIRECTION('',(1.,0.,0.));
#7455=DIRECTION('center_axis',(0.,1.,0.));
#7456=DIRECTION('ref_axis',(1.,0.,0.));
#7457=DIRECTION('',(-0.0523359562429438,0.,-0.998629534754574));
#7458=DIRECTION('',(-1.,0.,0.));
#7459=DIRECTION('',(0.0523359562429438,0.,0.998629534754574));
#7460=DIRECTION('',(-1.,0.,0.));
#7461=DIRECTION('center_axis',(0.,1.,0.));
#7462=DIRECTION('ref_axis',(1.,0.,0.));
#7463=DIRECTION('',(0.,0.,1.));
#7464=DIRECTION('',(-1.,0.,0.));
#7465=DIRECTION('',(0.,0.,-1.));
#7466=DIRECTION('',(-1.,0.,0.));
#7467=DIRECTION('center_axis',(0.,1.,0.));
#7468=DIRECTION('ref_axis',(1.,0.,0.));
#7469=DIRECTION('',(0.,0.,1.));
#7470=DIRECTION('',(-1.,0.,0.));
#7471=DIRECTION('',(0.,0.,-1.));
#7472=DIRECTION('',(-1.,0.,0.));
#7473=DIRECTION('center_axis',(0.,0.,1.));
#7474=DIRECTION('ref_axis',(1.,0.,0.));
#7475=DIRECTION('center_axis',(0.,0.,1.));
#7476=DIRECTION('ref_axis',(1.,0.,0.));
#7477=DIRECTION('center_axis',(0.,0.,1.));
#7478=DIRECTION('ref_axis',(1.,0.,0.));
#7479=DIRECTION('center_axis',(0.,0.,1.));
#7480=DIRECTION('ref_axis',(1.,0.,0.));
#7481=DIRECTION('center_axis',(0.,0.,1.));
#7482=DIRECTION('ref_axis',(1.,0.,0.));
#7483=DIRECTION('',(0.,1.,0.));
#7484=DIRECTION('',(0.,-1.,0.));
#7485=DIRECTION('center_axis',(0.,0.,1.));
#7486=DIRECTION('ref_axis',(1.,0.,0.));
#7487=DIRECTION('',(0.,-1.,0.));
#7488=DIRECTION('',(0.,1.,0.));
#7489=DIRECTION('center_axis',(0.,0.,1.));
#7490=DIRECTION('ref_axis',(1.,0.,0.));
#7491=DIRECTION('',(0.,-1.,0.));
#7492=DIRECTION('',(0.,1.,0.));
#7493=DIRECTION('center_axis',(0.,0.,1.));
#7494=DIRECTION('ref_axis',(1.,0.,0.));
#7495=DIRECTION('',(0.,-1.,0.));
#7496=DIRECTION('',(-1.,0.,0.));
#7497=DIRECTION('',(0.,1.,0.));
#7498=DIRECTION('center_axis',(0.,1.,0.));
#7499=DIRECTION('ref_axis',(1.,0.,0.));
#7500=DIRECTION('',(0.,0.,1.));
#7501=DIRECTION('',(-1.,0.,0.));
#7502=DIRECTION('',(0.,0.,-1.));
#7503=DIRECTION('center_axis',(-1.,0.,0.));
#7504=DIRECTION('ref_axis',(0.,-1.,0.));
#7505=DIRECTION('',(0.,-1.,0.));
#7506=DIRECTION('center_axis',(1.,0.,0.));
#7507=DIRECTION('ref_axis',(0.,1.,0.));
#7508=DIRECTION('',(0.,1.,0.));
#7509=DIRECTION('',(0.,1.,0.));
#7510=DIRECTION('center_axis',(1.,0.,0.));
#7511=DIRECTION('ref_axis',(0.,1.,0.));
#7512=DIRECTION('',(0.,1.,0.));
#7513=DIRECTION('',(0.,1.,1.13946463231163E-19));
#7514=DIRECTION('',(0.,1.,0.));
#7515=DIRECTION('center_axis',(1.,0.,0.));
#7516=DIRECTION('ref_axis',(0.,1.,0.));
#7517=DIRECTION('',(0.,1.,0.));
#7518=DIRECTION('',(0.,1.,1.13946463231163E-19));
#7519=DIRECTION('',(0.,1.,0.));
#7520=DIRECTION('center_axis',(0.998629534754574,0.,-0.0523359562429438));
#7521=DIRECTION('ref_axis',(-0.0523359562429438,0.,-0.998629534754574));
#7522=DIRECTION('',(0.,-1.,0.));
#7523=DIRECTION('',(-5.97168109510197E-21,-1.,-1.13946463231163E-19));
#7524=DIRECTION('',(0.,-1.,0.));
#7525=DIRECTION('center_axis',(0.,0.,1.));
#7526=DIRECTION('ref_axis',(1.,0.,0.));
#7527=DIRECTION('',(0.,-1.,0.));
#7528=DIRECTION('',(0.,-1.,0.));
#7529=DIRECTION('',(0.,-1.,0.));
#7530=DIRECTION('',(0.,1.,0.));
#7531=DIRECTION('',(0.,-1.,0.));
#7532=DIRECTION('',(0.,1.,0.));
#7533=DIRECTION('',(0.,-1.,0.));
#7534=DIRECTION('',(0.,-1.,0.));
#7535=DIRECTION('',(0.,-1.,0.));
#7536=DIRECTION('',(0.,1.,0.));
#7537=DIRECTION('',(0.,1.,0.));
#7538=DIRECTION('center_axis',(0.,0.,1.));
#7539=DIRECTION('ref_axis',(1.,0.,0.));
#7540=DIRECTION('',(0.,0.,-1.));
#7541=DIRECTION('center_axis',(0.,0.,1.));
#7542=DIRECTION('ref_axis',(1.,0.,0.));
#7543=DIRECTION('center_axis',(4.10828654779316E-33,-1.13946463231163E-19,
1.));
#7544=DIRECTION('ref_axis',(1.,0.,0.));
#7545=DIRECTION('',(0.,0.,-1.));
#7546=DIRECTION('center_axis',(1.,0.,0.));
#7547=DIRECTION('ref_axis',(0.,1.,0.));
#7548=DIRECTION('',(0.,1.,1.13946463231163E-19));
#7549=DIRECTION('center_axis',(0.99852593895705,0.0542765992849681,9.38276897523041E-9));
#7550=DIRECTION('ref_axis',(0.0541946171271057,-0.99701772369063,0.0549418066794405));
#7551=DIRECTION('center_axis',(4.10828654779316E-33,-1.13946463231163E-19,
1.));
#7552=DIRECTION('ref_axis',(1.,0.,-4.10828654779316E-33));
#7553=DIRECTION('',(5.97168109510217E-21,-1.,-1.13946463231163E-19));
#7554=DIRECTION('center_axis',(-1.,0.,0.));
#7555=DIRECTION('ref_axis',(0.,-1.,0.));
#7556=DIRECTION('',(0.,-1.,-1.13946463231163E-19));
#7557=DIRECTION('center_axis',(4.10828654779316E-33,-1.13946463231163E-19,
1.));
#7558=DIRECTION('ref_axis',(1.,0.,-4.10828654779316E-33));
#7559=DIRECTION('center_axis',(-1.,0.,0.));
#7560=DIRECTION('ref_axis',(0.,-1.,0.));
#7561=DIRECTION('',(0.,-1.,-1.13946463231163E-19));
#7562=DIRECTION('center_axis',(4.10828654779316E-33,-1.13946463231163E-19,
1.));
#7563=DIRECTION('ref_axis',(1.,0.,-4.10828654779316E-33));
#7564=DIRECTION('center_axis',(-1.,0.,0.));
#7565=DIRECTION('ref_axis',(0.,-1.,0.));
#7566=DIRECTION('',(0.,-1.,-1.13946463231163E-19));
#7567=DIRECTION('center_axis',(-0.996961060527779,0.0779015005717205,0.));
#7568=DIRECTION('ref_axis',(0.,0.,1.));
#7569=DIRECTION('center_axis',(4.10828654779316E-33,-1.13946463231163E-19,
1.));
#7570=DIRECTION('ref_axis',(1.,0.,-4.10828654779316E-33));
#7571=DIRECTION('',(5.97168109510197E-21,1.,1.13946463231163E-19));
#7572=DIRECTION('center_axis',(-0.996961060527779,-0.0779015005717276,-4.485055189269E-15));
#7573=DIRECTION('ref_axis',(-0.0777791112471086,0.995394757055134,0.0560329142626144));
#7574=DIRECTION('center_axis',(-0.377317868652411,-0.840644185582845,0.388521015186253));
#7575=DIRECTION('ref_axis',(-0.58566693710526,0.541587807512093,0.603056287203763));
#7576=DIRECTION('center_axis',(7.41164423166535E-16,1.,0.));
#7577=DIRECTION('ref_axis',(0.,0.,1.));
#7578=DIRECTION('center_axis',(0.0522650005536027,-0.0520548592672972,0.997275619547472));
#7579=DIRECTION('ref_axis',(-0.998629534754574,7.40148683083438E-16,0.0523359562429445));
#7580=DIRECTION('center_axis',(0.376559988603802,-0.837471124372148,0.396036224133039));
#7581=DIRECTION('ref_axis',(0.577069986161316,0.546481578685729,0.606916893181374));
#7582=DIRECTION('center_axis',(0.998525938475037,-0.0542766081525538,0.));
#7583=DIRECTION('ref_axis',(0.,0.,1.));
#7584=DIRECTION('center_axis',(-0.0522648366634829,-0.0521149007022807,
0.997272492337641));
#7585=DIRECTION('ref_axis',(0.0541946171271058,0.99701772369063,0.0549418066794413));
#7586=DIRECTION('center_axis',(5.32220538281047E-11,1.,-1.01553728389566E-9));
#7587=DIRECTION('ref_axis',(0.998629534754574,0.,0.0523359562429456));
#7588=DIRECTION('center_axis',(0.37731786865241,-0.840644185582843,-0.388521015186259));
#7589=DIRECTION('ref_axis',(-0.585666937105255,-0.541587807512096,0.603056287203765));
#7590=DIRECTION('center_axis',(0.0522650005536027,0.0520548592672965,0.997275619547472));
#7591=DIRECTION('ref_axis',(-0.0777791112471059,-0.995394757055134,0.0560329142626137));
#7592=DIRECTION('center_axis',(0.,-1.,0.));
#7593=DIRECTION('ref_axis',(-0.998629534754574,0.,0.0523359562429439));
#7594=DIRECTION('center_axis',(5.97168109510197E-21,1.,1.13946463231163E-19));
#7595=DIRECTION('ref_axis',(-0.688354575693753,0.,0.725374371012288));
#7596=DIRECTION('center_axis',(-0.376559987018669,-0.837471124206646,-0.396036225990193));
#7597=DIRECTION('ref_axis',(0.577069983350267,-0.54648157893936,0.606916895625808));
#7598=DIRECTION('center_axis',(-0.0522648366634817,0.0521149007022785,0.997272492337641));
#7599=DIRECTION('ref_axis',(0.998629534754574,0.,0.052335956242946));
#7600=DIRECTION('center_axis',(1.01693095242295E-9,-1.,0.));
#7601=DIRECTION('ref_axis',(0.,0.,1.));
#7602=DIRECTION('center_axis',(5.97168109510217E-21,-1.,-1.13946463231163E-19));
#7603=DIRECTION('ref_axis',(0.688354575693753,0.,0.725374371012289));
#7604=DIRECTION('',(-5.97168109510217E-21,1.,1.13946463231163E-19));
#7605=DIRECTION('center_axis',(-0.998629534754574,0.,-0.0523359562429455));
#7606=DIRECTION('ref_axis',(-0.0523359562429455,0.,0.998629534754574));
#7607=DIRECTION('center_axis',(-0.377317868652411,-0.840644185582845,0.388521015186254));
#7608=DIRECTION('ref_axis',(-0.585666937105261,0.541587807512092,0.603056287203763));
#7609=DIRECTION('center_axis',(7.41164423166535E-16,1.,0.));
#7610=DIRECTION('ref_axis',(0.,0.,1.));
#7611=DIRECTION('center_axis',(-0.996961060527779,-0.0779015005717276,-4.485055189269E-15));
#7612=DIRECTION('ref_axis',(-0.0777791112471086,0.995394757055134,0.0560329142626144));
#7613=DIRECTION('center_axis',(0.0522650005536027,-0.0520548592672972,0.997275619547472));
#7614=DIRECTION('ref_axis',(-0.998629534754574,7.40148683083438E-16,0.0523359562429445));
#7615=DIRECTION('center_axis',(0.376559988603802,-0.837471124372148,0.396036224133039));
#7616=DIRECTION('ref_axis',(0.577069986161311,0.546481578685732,0.606916893181376));
#7617=DIRECTION('center_axis',(0.998525938475037,-0.0542766081525538,0.));
#7618=DIRECTION('ref_axis',(0.,0.,1.));
#7619=DIRECTION('center_axis',(5.32220538281047E-11,1.,-1.01553728389566E-9));
#7620=DIRECTION('ref_axis',(0.998629534754574,0.,0.0523359562429456));
#7621=DIRECTION('center_axis',(-0.0522648366634829,-0.0521149007022807,
0.997272492337641));
#7622=DIRECTION('ref_axis',(0.0541946171271058,0.99701772369063,0.0549418066794413));
#7623=DIRECTION('center_axis',(0.37731786865241,-0.840644185582843,-0.388521015186259));
#7624=DIRECTION('ref_axis',(-0.585666937105255,-0.541587807512095,0.603056287203766));
#7625=DIRECTION('center_axis',(-0.996961060527779,0.0779015005717205,0.));
#7626=DIRECTION('ref_axis',(0.,0.,1.));
#7627=DIRECTION('center_axis',(0.,-1.,0.));
#7628=DIRECTION('ref_axis',(-0.998629534754574,0.,0.0523359562429439));
#7629=DIRECTION('center_axis',(0.0522650005536027,0.0520548592672965,0.997275619547472));
#7630=DIRECTION('ref_axis',(-0.0777791112471059,-0.995394757055134,0.0560329142626137));
#7631=DIRECTION('center_axis',(5.97168109510197E-21,1.,1.13946463231163E-19));
#7632=DIRECTION('ref_axis',(-0.688354575693753,0.,0.725374371012289));
#7633=DIRECTION('',(-5.97168109510197E-21,-1.,-1.13946463231163E-19));
#7634=DIRECTION('',(5.97168109510197E-21,1.,1.13946463231163E-19));
#7635=DIRECTION('center_axis',(-0.376559987018669,-0.837471124206646,-0.396036225990194));
#7636=DIRECTION('ref_axis',(0.577069983350267,-0.546481578939359,0.606916895625808));
#7637=DIRECTION('center_axis',(-0.0522648366634817,0.0521149007022785,0.997272492337641));
#7638=DIRECTION('ref_axis',(0.998629534754574,0.,0.052335956242946));
#7639=DIRECTION('center_axis',(1.01693095242295E-9,-1.,0.));
#7640=DIRECTION('ref_axis',(0.,0.,1.));
#7641=DIRECTION('center_axis',(0.99852593895705,0.0542765992849681,9.38276897523041E-9));
#7642=DIRECTION('ref_axis',(0.0541946171271057,-0.99701772369063,0.0549418066794405));
#7643=DIRECTION('center_axis',(5.97168109510217E-21,-1.,-1.13946463231163E-19));
#7644=DIRECTION('ref_axis',(0.688354575693753,0.,0.725374371012289));
#7645=DIRECTION('',(-5.97168109510217E-21,1.,1.13946463231163E-19));
#7646=DIRECTION('',(5.97168109510217E-21,-1.,-1.13946463231163E-19));
#7647=DIRECTION('center_axis',(0.998629534754574,0.,-0.0523359562429438));
#7648=DIRECTION('ref_axis',(-0.0523359562429438,0.,-0.998629534754574));
#7649=DIRECTION('center_axis',(4.10828654779316E-33,-1.13946463231163E-19,
1.));
#7650=DIRECTION('ref_axis',(1.,0.,-4.10828654779316E-33));
#7651=DIRECTION('center_axis',(-0.998629534754574,0.,-0.0523359562429455));
#7652=DIRECTION('ref_axis',(-0.0523359562429455,0.,0.998629534754574));
#8711=CARTESIAN_POINT('',(0.,0.,0.));
#8712=CARTESIAN_POINT('Origin',(8.1,-1.,0.7));
#8713=CARTESIAN_POINT('',(7.94916965151797,-1.19937453693185,0.7));
#8714=CARTESIAN_POINT('',(8.26514540988519,-1.18768855477586,0.7));
#8715=CARTESIAN_POINT('Ctrl Pts',(7.94916965151797,-1.19937453693185,0.7));
#8716=CARTESIAN_POINT('Ctrl Pts',(7.97160858810976,-1.21634998764782,0.7));
#8717=CARTESIAN_POINT('Ctrl Pts',(7.99739856866269,-1.22989011121344,0.69528529300377));
#8718=CARTESIAN_POINT('Ctrl Pts',(8.03944443766207,-1.24298414277179,0.688517705185315));
#8719=CARTESIAN_POINT('Ctrl Pts',(8.05362924383607,-1.24609346022897,0.686388676887586));
#8720=CARTESIAN_POINT('Ctrl Pts',(8.075506183533,-1.24890990228851,0.684139035126277));
#8721=CARTESIAN_POINT('Ctrl Pts',(8.08297567221474,-1.24953307703463,0.683546226354886));
#8722=CARTESIAN_POINT('Ctrl Pts',(8.0940066533036,-1.24995288972095,0.68299521602547));
#8723=CARTESIAN_POINT('Ctrl Pts',(8.09752287926269,-1.25001251279495,0.68286729538075));
#8724=CARTESIAN_POINT('Ctrl Pts',(8.10293413375911,-1.249989933108,0.682747340264197));
#8725=CARTESIAN_POINT('Ctrl Pts',(8.10482478940148,-1.24996059450444,0.682719828470948));
#8726=CARTESIAN_POINT('Ctrl Pts',(8.10828546792054,-1.24986760009171,0.682696100760705));
#8727=CARTESIAN_POINT('Ctrl Pts',(8.10985478687837,-1.24981062779486,0.682695370268813));
#8728=CARTESIAN_POINT('Ctrl Pts',(8.11326464342549,-1.24965465239671,0.682715595753076));
#8729=CARTESIAN_POINT('Ctrl Pts',(8.11510409202247,-1.2495501177419,0.682740330911594));
#8730=CARTESIAN_POINT('Ctrl Pts',(8.12014207260669,-1.24920790966494,0.682845651127781));
#8731=CARTESIAN_POINT('Ctrl Pts',(8.12333423895876,-1.24892926854386,0.682953992816581));
#8732=CARTESIAN_POINT('Ctrl Pts',(8.139194120874,-1.2472372768871,0.683691668462565));
#8733=CARTESIAN_POINT('Ctrl Pts',(8.15164141295685,-1.2449338270761,0.684918799511701));
#8734=CARTESIAN_POINT('Ctrl Pts',(8.19196937649467,-1.23428099896052,0.690212518998986));
#8735=CARTESIAN_POINT('Ctrl Pts',(8.21811504697062,-1.22213176592155,0.695755006185672));
#8736=CARTESIAN_POINT('Ctrl Pts',(8.24962874265135,-1.20052913769617,0.699397421419897));
#8737=CARTESIAN_POINT('Ctrl Pts',(8.25758631484639,-1.19433973204149,0.7));
#8738=CARTESIAN_POINT('Ctrl Pts',(8.26514540988519,-1.18768855477586,0.7));
#8739=CARTESIAN_POINT('Origin',(8.1,-1.,0.7));
#8740=CARTESIAN_POINT('Origin',(2.7,1.,0.7));
#8741=CARTESIAN_POINT('',(2.8076286513348,1.22564590451442,0.7));
#8742=CARTESIAN_POINT('',(2.57739843082973,1.21787348447435,0.7));
#8743=CARTESIAN_POINT('Ctrl Pts',(2.80762864495888,1.22564590575571,0.7));
#8744=CARTESIAN_POINT('Ctrl Pts',(2.78743249310418,1.23527907171202,0.7));
#8745=CARTESIAN_POINT('Ctrl Pts',(2.76507271635938,1.24261561512899,0.698430289974852));
#8746=CARTESIAN_POINT('Ctrl Pts',(2.73219941643314,1.24807722603274,0.696876198609429));
#8747=CARTESIAN_POINT('Ctrl Pts',(2.72335305886828,1.24906618730719,0.696525251810408));
#8748=CARTESIAN_POINT('Ctrl Pts',(2.71018695034311,1.24982905432238,0.696188910804419));
#8749=CARTESIAN_POINT('Ctrl Pts',(2.70590779780308,1.24996687586326,0.696107915309552));
#8750=CARTESIAN_POINT('Ctrl Pts',(2.69921702211412,1.25001037316246,0.696030339680738));
#8751=CARTESIAN_POINT('Ctrl Pts',(2.69680890442544,1.24999123464332,0.696012302673685));
#8752=CARTESIAN_POINT('Ctrl Pts',(2.69234597975348,1.24989125947742,0.695997601992606));
#8753=CARTESIAN_POINT('Ctrl Pts',(2.69029169500035,1.24981988388707,0.69599819279703));
#8754=CARTESIAN_POINT('Ctrl Pts',(2.6857660481318,1.24960673159635,0.696015705561832));
#8755=CARTESIAN_POINT('Ctrl Pts',(2.68329599580702,1.24945360531346,0.696035938105249));
#8756=CARTESIAN_POINT('Ctrl Pts',(2.67625328071593,1.24891193026541,0.696123377063474));
#8757=CARTESIAN_POINT('Ctrl Pts',(2.67169109188753,1.24843439216159,0.696216059649547));
#8758=CARTESIAN_POINT('Ctrl Pts',(2.64765560351845,1.24524789167778,0.696873729305584));
#8759=CARTESIAN_POINT('Ctrl Pts',(2.62857598726268,1.24037162800668,0.698048768812303));
#8760=CARTESIAN_POINT('Ctrl Pts',(2.59902076831046,1.22902239593109,0.699541037747764));
#8761=CARTESIAN_POINT('Ctrl Pts',(2.58799157881597,1.22383445108162,0.7));
#8762=CARTESIAN_POINT('Ctrl Pts',(2.57739843082979,1.21787348447436,0.7));
#8763=CARTESIAN_POINT('Origin',(2.7,1.,0.7));
#8764=CARTESIAN_POINT('Origin',(2.7,-1.,0.7));
#8765=CARTESIAN_POINT('',(2.57739843082979,-1.21787348447436,0.7));
#8766=CARTESIAN_POINT('',(2.80762864495888,-1.22564590575571,0.7));
#8767=CARTESIAN_POINT('Ctrl Pts',(2.57739843082979,-1.21787348447436,0.7));
#8768=CARTESIAN_POINT('Ctrl Pts',(2.59689796709118,-1.22884624579732,0.7));
#8769=CARTESIAN_POINT('Ctrl Pts',(2.61871070177046,-1.23767364961455,0.698430520021629));
#8770=CARTESIAN_POINT('Ctrl Pts',(2.6511387549791,-1.24533993869645,0.696876447160353));
#8771=CARTESIAN_POINT('Ctrl Pts',(2.65989793055836,-1.24692336726652,0.696525471319567));
#8772=CARTESIAN_POINT('Ctrl Pts',(2.67298219502323,-1.24857266139659,0.696189053183015));
#8773=CARTESIAN_POINT('Ctrl Pts',(2.67724223626036,-1.24899884484677,0.696108027479433));
#8774=CARTESIAN_POINT('Ctrl Pts',(2.68391475503581,-1.24949361628703,0.696030400846995));
#8775=CARTESIAN_POINT('Ctrl Pts',(2.68631866330158,-1.24963697932539,0.69601234479389));
#8776=CARTESIAN_POINT('Ctrl Pts',(2.69077815115796,-1.24983831390468,0.695997608323079));
#8777=CARTESIAN_POINT('Ctrl Pts',(2.69283257145917,-1.24990568929416,0.695998182544699));
#8778=CARTESIAN_POINT('Ctrl Pts',(2.69736230434386,-1.24999833696454,0.696015659042177));
#8779=CARTESIAN_POINT('Ctrl Pts',(2.69983707579759,-1.25001219669429,0.696035872086962));
#8780=CARTESIAN_POINT('Ctrl Pts',(2.70690037992806,-1.24994687665095,0.696123257636812));
#8781=CARTESIAN_POINT('Ctrl Pts',(2.71148446565418,-1.24977820005943,0.696215908504701));
#8782=CARTESIAN_POINT('Ctrl Pts',(2.73568105999059,-1.24822038288304,0.696873447340259));
#8783=CARTESIAN_POINT('Ctrl Pts',(2.75504695022812,-1.24464213141243,0.698048515307351));
#8784=CARTESIAN_POINT('Ctrl Pts',(2.78530198112344,-1.2353118289445,0.699540950501024));
#8785=CARTESIAN_POINT('Ctrl Pts',(2.79665680001786,-1.23087925931356,0.7));
#8786=CARTESIAN_POINT('Ctrl Pts',(2.80762864495888,-1.22564590575571,0.7));
#8787=CARTESIAN_POINT('Origin',(2.7,-1.,0.7));
#8788=CARTESIAN_POINT('Origin',(8.1,1.,0.7));
#8789=CARTESIAN_POINT('',(8.26514540988519,1.18768855477586,0.7));
#8790=CARTESIAN_POINT('',(7.94916965249954,1.19937453719419,0.7));
#8791=CARTESIAN_POINT('Ctrl Pts',(8.26514540988519,1.18768855477586,0.7));
#8792=CARTESIAN_POINT('Ctrl Pts',(8.24402114884725,1.20627559516199,0.7));
#8793=CARTESIAN_POINT('Ctrl Pts',(8.21930102059268,1.22168408824046,0.695284768760077));
#8794=CARTESIAN_POINT('Ctrl Pts',(8.17833936508797,1.23784683595578,0.688517484674842));
#8795=CARTESIAN_POINT('Ctrl Pts',(8.16442627443898,1.24199461640617,0.686388979601913));
#8796=CARTESIAN_POINT('Ctrl Pts',(8.14282164862934,1.24641910835203,0.684139556285851));
#8797=CARTESIAN_POINT('Ctrl Pts',(8.13541969045672,1.24759243465272,0.683546718614312));
#8798=CARTESIAN_POINT('Ctrl Pts',(8.12445132655127,1.24882623938238,0.682995554842566));
#8799=CARTESIAN_POINT('Ctrl Pts',(8.12094947916695,1.24914555886372,0.68286756899844));
#8800=CARTESIAN_POINT('Ctrl Pts',(8.11555178799172,1.24952297970176,0.682747494033431));
#8801=CARTESIAN_POINT('Ctrl Pts',(8.11366421100955,1.24963346420394,0.682719937279798));
#8802=CARTESIAN_POINT('Ctrl Pts',(8.11020620287515,1.24979651712922,0.682696124556263));
#8803=CARTESIAN_POINT('Ctrl Pts',(8.10863696767328,1.24985569708818,0.682695355189016));
#8804=CARTESIAN_POINT('Ctrl Pts',(8.10522484403353,1.249952190393,0.682715496638402));
#8805=CARTESIAN_POINT('Ctrl Pts',(8.10338263267786,1.24998390529834,0.682740187713169));
#8806=CARTESIAN_POINT('Ctrl Pts',(8.09833277498968,1.25001501472208,0.682845394223802));
#8807=CARTESIAN_POINT('Ctrl Pts',(8.09512844909059,1.24997307323179,0.682953673497893));
#8808=CARTESIAN_POINT('Ctrl Pts',(8.07918314804204,1.24945780552822,0.683691186949858));
#8809=CARTESIAN_POINT('Ctrl Pts',(8.06659630270856,1.24808001426183,0.684918585227095));
#8810=CARTESIAN_POINT('Ctrl Pts',(8.02558960427868,1.24043495378573,0.69021260546313));
#8811=CARTESIAN_POINT('Ctrl Pts',(7.9986188553413,1.2302509517108,0.695754623970086));
#8812=CARTESIAN_POINT('Ctrl Pts',(7.96559475436581,1.21103543221342,0.69939729083119));
#8813=CARTESIAN_POINT('Ctrl Pts',(7.95720051358587,1.20545002552208,0.7));
#8814=CARTESIAN_POINT('Ctrl Pts',(7.94916965151797,1.19937453693185,0.7));
#8815=CARTESIAN_POINT('Origin',(8.1,1.,0.7));
#8816=CARTESIAN_POINT('Ctrl Pts',(1.1,1.14549341399196,0.7));
#8817=CARTESIAN_POINT('Ctrl Pts',(1.89984199608574,1.1957170361627,0.7));
#8818=CARTESIAN_POINT('Ctrl Pts',(2.70080437300401,1.2273695200909,0.7));
#8819=CARTESIAN_POINT('Ctrl Pts',(3.50204003610941,1.24374118183538,0.7));
#8820=CARTESIAN_POINT('Ctrl Pts',(1.09819048660397,1.17431102498992,0.7));
#8821=CARTESIAN_POINT('Ctrl Pts',(1.89847848223077,1.22458382597074,0.70000077422621));
#8822=CARTESIAN_POINT('Ctrl Pts',(2.69984520196781,1.25626413437997,0.699999727319846));
#8823=CARTESIAN_POINT('Ctrl Pts',(3.50144932661635,1.27265074030048,0.700000000000001));
#8824=CARTESIAN_POINT('Ctrl Pts',(1.09505363188407,1.22426736091617,0.676703190608825));
#8825=CARTESIAN_POINT('Ctrl Pts',(1.89610976425884,1.27462253270773,0.67666760713801));
#8826=CARTESIAN_POINT('Ctrl Pts',(2.69818680938115,1.3063522351595,0.67664530655333));
#8827=CARTESIAN_POINT('Ctrl Pts',(3.50042536655637,1.322763754511,0.676632802377821));
#8828=CARTESIAN_POINT('Ctrl Pts',(1.09381704710221,1.24396073223232,0.627109609335854));
#8829=CARTESIAN_POINT('Ctrl Pts',(1.89518106151152,1.29430885982199,0.62701751976321));
#8830=CARTESIAN_POINT('Ctrl Pts',(2.69753328610131,1.32603127467068,0.626959208652505));
#8831=CARTESIAN_POINT('Ctrl Pts',(3.50002334924346,1.34243864233338,0.626926882269943));
#8832=CARTESIAN_POINT('Ctrl Pts',(1.09374258853658,1.24514653057163,0.605486452199395));
#8833=CARTESIAN_POINT('Ctrl Pts',(1.89512529323683,1.29547288309274,0.605377720397184));
#8834=CARTESIAN_POINT('Ctrl Pts',(2.69749615303001,1.32718177535833,0.605308474776761));
#8835=CARTESIAN_POINT('Ctrl Pts',(3.5,1.34358136363184,0.605270327458635));
#8836=CARTESIAN_POINT('',(1.1,1.14549341399195,0.7));
#8837=CARTESIAN_POINT('Ctrl Pts',(1.1,1.14549341399196,0.7));
#8838=CARTESIAN_POINT('Ctrl Pts',(1.59210562457523,1.17639367564078,0.7));
#8839=CARTESIAN_POINT('Ctrl Pts',(2.08463535466703,1.20026407570248,0.7));
#8840=CARTESIAN_POINT('Ctrl Pts',(2.57739190516306,1.2178709162388,0.7));
#8841=CARTESIAN_POINT('',(1.1,1.24553911298206,0.605485603995113));
#8842=CARTESIAN_POINT('Ctrl Pts',(1.1,1.14549341399196,0.7));
#8843=CARTESIAN_POINT('Ctrl Pts',(1.1,1.15341616150799,0.7));
#8844=CARTESIAN_POINT('Ctrl Pts',(1.1000012416168,1.16127613060545,0.699006361583129));
#8845=CARTESIAN_POINT('Ctrl Pts',(1.10000231308998,1.16893252943985,0.697119293189023));
#8846=CARTESIAN_POINT('Ctrl Pts',(1.10000291357081,1.17322337016277,0.696061732044743));
#8847=CARTESIAN_POINT('Ctrl Pts',(1.10000345673767,1.17745032641463,0.694722535963768));
#8848=CARTESIAN_POINT('Ctrl Pts',(1.10000379529503,1.18158693416151,0.693112479763539));
#8849=CARTESIAN_POINT('Ctrl Pts',(1.1000044034764,1.18901789868739,0.690220189452084));
#8850=CARTESIAN_POINT('Ctrl Pts',(1.1000042334852,1.19607766167095,0.686488065947256));
#8851=CARTESIAN_POINT('Ctrl Pts',(1.10000339376692,1.2026196529327,0.681996646156542));
#8852=CARTESIAN_POINT('Ctrl Pts',(1.10000293249552,1.20621327895058,0.67952943359521));
#8853=CARTESIAN_POINT('Ctrl Pts',(1.10000228571683,1.20965039763183,0.676832226278619));
#8854=CARTESIAN_POINT('Ctrl Pts',(1.10000171524363,1.21290279159005,0.673912896410569));
#8855=CARTESIAN_POINT('Ctrl Pts',(1.10000115816795,1.2160788033717,0.671062126739188));
#8856=CARTESIAN_POINT('Ctrl Pts',(1.10000066850715,1.2190594221245,0.668016750164662));
#8857=CARTESIAN_POINT('Ctrl Pts',(1.10000067525152,1.22182202639256,0.664788091882127));
#8858=CARTESIAN_POINT('Ctrl Pts',(1.10000068775799,1.22694487635592,0.658801012170571));
#8859=CARTESIAN_POINT('Ctrl Pts',(1.10000222199399,1.23132099043293,0.652185071179834));
#8860=CARTESIAN_POINT('Ctrl Pts',(1.10000276904041,1.23488987417606,0.64510534613808));
#8861=CARTESIAN_POINT('Ctrl Pts',(1.10000282439334,1.23525099193115,0.644388983656765));
#8862=CARTESIAN_POINT('Ctrl Pts',(1.10000287212626,1.23560380546488,0.64366785367332));
#8863=CARTESIAN_POINT('Ctrl Pts',(1.10000291138002,1.23594822450451,0.642942116631622));
#8864=CARTESIAN_POINT('Ctrl Pts',(1.10000329911404,1.23935026814133,0.635773555081239));
#8865=CARTESIAN_POINT('Ctrl Pts',(1.10000258010782,1.24189771450306,0.628240464257889));
#8866=CARTESIAN_POINT('Ctrl Pts',(1.10000149084855,1.24353681278199,0.620511076118615));
#8867=CARTESIAN_POINT('Ctrl Pts',(1.10000079446814,1.24458471384188,0.615569557890241));
#8868=CARTESIAN_POINT('Ctrl Pts',(1.10000000111128,1.24526049271905,0.610547146027233));
#8869=CARTESIAN_POINT('Ctrl Pts',(1.09999999916631,1.24553911263843,0.605485603997432));
#8870=CARTESIAN_POINT('',(3.5,1.34358136363184,0.605270327458635));
#8871=CARTESIAN_POINT('Ctrl Pts',(3.5,1.34358136363184,0.605270327458635));
#8872=CARTESIAN_POINT('Ctrl Pts',(2.6995848679345,1.32722445934619,0.605308375488923));
#8873=CARTESIAN_POINT('Ctrl Pts',(1.89930203168261,1.29563783986497,0.605377360150118));
#8874=CARTESIAN_POINT('Ctrl Pts',(1.09999999916631,1.24553911263843,0.605485603997431));
#8875=CARTESIAN_POINT('',(3.5,1.24369946473792,0.7));
#8876=CARTESIAN_POINT('Ctrl Pts',(3.5,1.34358136363184,0.605270327458635));
#8877=CARTESIAN_POINT('Ctrl Pts',(3.5,1.34316359984937,0.613184373088104));
#8878=CARTESIAN_POINT('Ctrl Pts',(3.50000057901142,1.34177887744868,0.621008021569537));
#8879=CARTESIAN_POINT('Ctrl Pts',(3.50000082863025,1.33951086762262,0.628580534231506));
#8880=CARTESIAN_POINT('Ctrl Pts',(3.50000096811,1.33824356956914,0.632811834486987));
#8881=CARTESIAN_POINT('Ctrl Pts',(3.50000102536574,1.33669948631919,0.636964759527324));
#8882=CARTESIAN_POINT('Ctrl Pts',(3.50000098105742,1.334886463945,0.641009258704104));
#8883=CARTESIAN_POINT('Ctrl Pts',(3.50000090179773,1.3316432906201,0.648244145614236));
#8884=CARTESIAN_POINT('Ctrl Pts',(3.50000044940971,1.3275777080273,0.655054131048541));
#8885=CARTESIAN_POINT('Ctrl Pts',(3.50000027423476,1.32275302640998,0.661275670751788));
#8886=CARTESIAN_POINT('Ctrl Pts',(3.50000024156065,1.32185311357394,0.66243612938574));
#8887=CARTESIAN_POINT('Ctrl Pts',(3.50000022115524,1.32092666334894,0.663576045687695));
#8888=CARTESIAN_POINT('Ctrl Pts',(3.50000022069074,1.31997391848392,0.664694242102532));
#8889=CARTESIAN_POINT('Ctrl Pts',(3.50000021976176,1.31806844339147,0.666930617752677));
#8890=CARTESIAN_POINT('Ctrl Pts',(3.50000029790302,1.31605782519,0.669080165434128));
#8891=CARTESIAN_POINT('Ctrl Pts',(3.50000040488465,1.31394946763378,0.671139079687271));
#8892=CARTESIAN_POINT('Ctrl Pts',(3.50000069329649,1.3082655455861,0.6766897075128));
#8893=CARTESIAN_POINT('Ctrl Pts',(3.5000011432336,1.30193818666762,0.681521899278667));
#8894=CARTESIAN_POINT('Ctrl Pts',(3.50000129797765,1.29513115062548,0.68558123547136));
#8895=CARTESIAN_POINT('Ctrl Pts',(3.50000139624096,1.2908086457691,0.688158936000333));
#8896=CARTESIAN_POINT('Ctrl Pts',(3.50000139493488,1.28629176508013,0.690424313967808));
#8897=CARTESIAN_POINT('Ctrl Pts',(3.50000129141552,1.28161680488022,0.692354162840695));
#8898=CARTESIAN_POINT('Ctrl Pts',(3.50000112941005,1.27430059661786,0.695374333209024));
#8899=CARTESIAN_POINT('Ctrl Pts',(3.5000007162179,1.26668229982361,0.697540280949125));
#8900=CARTESIAN_POINT('Ctrl Pts',(3.50000038344698,1.25890895215876,0.698782355543395));
#8901=CARTESIAN_POINT('Ctrl Pts',(3.50000016866387,1.25389173534334,0.699584038140014));
#8902=CARTESIAN_POINT('Ctrl Pts',(3.4999999993056,1.24880933504677,0.69999999987784));
#8903=CARTESIAN_POINT('Ctrl Pts',(3.49999999991873,1.24369946470729,0.7));
#8904=CARTESIAN_POINT('Ctrl Pts',(2.80762377174497,1.22564400643366,0.7));
#8905=CARTESIAN_POINT('Ctrl Pts',(3.03837960601223,1.23298334400942,0.7));
#8906=CARTESIAN_POINT('Ctrl Pts',(3.26917843294065,1.23897560812206,0.7));
#8907=CARTESIAN_POINT('Ctrl Pts',(3.49999999991873,1.24369946470729,0.7));
#8908=CARTESIAN_POINT('Ctrl Pts',(7.29709043526678,1.22049830417059,0.7));
#8909=CARTESIAN_POINT('Ctrl Pts',(8.19846709497879,1.19422430779862,0.7));
#8910=CARTESIAN_POINT('Ctrl Pts',(9.09944331332256,1.15544418981837,0.7));
#8911=CARTESIAN_POINT('Ctrl Pts',(10.,1.10900986674273,0.7));
#8912=CARTESIAN_POINT('Ctrl Pts',(7.29793284700474,1.24939875264889,0.7));
#8913=CARTESIAN_POINT('Ctrl Pts',(8.19957769811722,1.22310890030201,0.699999704549177));
#8914=CARTESIAN_POINT('Ctrl Pts',(9.10076698492607,1.18430758604571,0.700000491839571));
#8915=CARTESIAN_POINT('Ctrl Pts',(10.0014871213396,1.13785139984992,0.7));
#8916=CARTESIAN_POINT('Ctrl Pts',(7.29939288958794,1.29948813715084,0.676630595533454));
#8917=CARTESIAN_POINT('Ctrl Pts',(8.20149954052228,1.27317186922949,0.676644146017132));
#8918=CARTESIAN_POINT('Ctrl Pts',(9.10306300621911,1.23433322993607,0.676664155483857));
#8919=CARTESIAN_POINT('Ctrl Pts',(10.0040646682326,1.18784086746588,0.676686753673613));
#8920=CARTESIAN_POINT('Ctrl Pts',(7.29996660609513,1.31917051289423,0.626939603849942));
#8921=CARTESIAN_POINT('Ctrl Pts',(8.20225661204673,1.29285896783792,0.626974637782525));
#8922=CARTESIAN_POINT('Ctrl Pts',(9.10396596140606,1.25402923300358,0.627026849623412));
#8923=CARTESIAN_POINT('Ctrl Pts',(10.0050807923581,1.20754778500352,0.627085325222079));
#8924=CARTESIAN_POINT('Ctrl Pts',(7.29999999953093,1.32031613471704,0.605285370449856));
#8925=CARTESIAN_POINT('Ctrl Pts',(8.20230020786565,1.29401302889245,0.605326714446839));
#8926=CARTESIAN_POINT('Ctrl Pts',(9.10401978846669,1.25519559703033,0.605388684776982));
#8927=CARTESIAN_POINT('Ctrl Pts',(10.0051416645797,1.20872835322339,0.605457722909465));
#8928=CARTESIAN_POINT('',(7.29999999989017,1.22041345054104,0.7));
#8929=CARTESIAN_POINT('Ctrl Pts',(7.29999999978094,1.22041345055303,0.7));
#8930=CARTESIAN_POINT('Ctrl Pts',(7.51641201913776,1.21409884615949,0.7));
#8931=CARTESIAN_POINT('Ctrl Pts',(7.73280095443524,1.20706364503479,0.7));
#8932=CARTESIAN_POINT('Ctrl Pts',(7.94916654146952,1.19937499621344,0.7));
#8933=CARTESIAN_POINT('',(7.29999999953133,1.3203161347307,0.605285370449834));
#8934=CARTESIAN_POINT('Ctrl Pts',(7.29999999989087,1.22041345054982,0.7));
#8935=CARTESIAN_POINT('Ctrl Pts',(7.30000000079355,1.22832360919786,0.699999999740221));
#8936=CARTESIAN_POINT('Ctrl Pts',(7.29999941101664,1.23617007614594,0.699006006469939));
#8937=CARTESIAN_POINT('Ctrl Pts',(7.29999889581476,1.24381267896118,0.697118889344366));
#8938=CARTESIAN_POINT('Ctrl Pts',(7.29999860583198,1.24811433880851,0.696056720321257));
#8939=CARTESIAN_POINT('Ctrl Pts',(7.29999834128398,1.25235147078274,0.694710570513598));
#8940=CARTESIAN_POINT('Ctrl Pts',(7.29999817264931,1.25649739217805,0.693091458416622));
#8941=CARTESIAN_POINT('Ctrl Pts',(7.29999787070862,1.26392067210813,0.690192435210923));
#8942=CARTESIAN_POINT('Ctrl Pts',(7.29999793286912,1.27097116792553,0.686452948287278));
#8943=CARTESIAN_POINT('Ctrl Pts',(7.2999983123982,1.27750284616821,0.681954753865011));
#8944=CARTESIAN_POINT('Ctrl Pts',(7.2999985213788,1.28109939299731,0.679477906983553));
#8945=CARTESIAN_POINT('Ctrl Pts',(7.29999881895966,1.28453837241868,0.676770138671336));
#8946=CARTESIAN_POINT('Ctrl Pts',(7.29999908362886,1.28779148632494,0.673839551409954));
#8947=CARTESIAN_POINT('Ctrl Pts',(7.29999934163235,1.29096267037196,0.670982771155867));
#8948=CARTESIAN_POINT('Ctrl Pts',(7.29999957112158,1.2939379836903,0.667931525418885));
#8949=CARTESIAN_POINT('Ctrl Pts',(7.29999957127586,1.29669488996436,0.664697318929259));
#8950=CARTESIAN_POINT('Ctrl Pts',(7.29999957156178,1.30180432468448,0.658703293276094));
#8951=CARTESIAN_POINT('Ctrl Pts',(7.29999886995656,1.30616650855536,0.652082235935803));
#8952=CARTESIAN_POINT('Ctrl Pts',(7.29999863193158,1.30972187224872,0.644999691185358));
#8953=CARTESIAN_POINT('Ctrl Pts',(7.29999860759325,1.31008541227461,0.644275492840527));
#8954=CARTESIAN_POINT('Ctrl Pts',(7.29999858692673,1.31044047656777,0.643546449710686));
#8955=CARTESIAN_POINT('Ctrl Pts',(7.29999857034625,1.31078697300061,0.642812727646596));
#8956=CARTESIAN_POINT('Ctrl Pts',(7.29999840819729,1.31417553742296,0.635637287305567));
#8957=CARTESIAN_POINT('Ctrl Pts',(7.29999876577208,1.31670951795567,0.628098908385918));
#8958=CARTESIAN_POINT('Ctrl Pts',(7.29999928780719,1.3183355664444,0.620365998324013));
#8959=CARTESIAN_POINT('Ctrl Pts',(7.29999962266353,1.3193785856694,0.615405768714856));
#8960=CARTESIAN_POINT('Ctrl Pts',(7.3,1.32004717656055,0.610364828659741));
#8961=CARTESIAN_POINT('Ctrl Pts',(7.3,1.32031613470337,0.605285370449877));
#8962=CARTESIAN_POINT('',(10.,1.20899340483173,0.605457329065657));
#8963=CARTESIAN_POINT('Ctrl Pts',(9.99999999968202,1.20899340489109,0.605457329065633));
#8964=CARTESIAN_POINT('Ctrl Pts',(9.10058974048747,1.25534320916473,0.605388449123016));
#8965=CARTESIAN_POINT('Ctrl Pts',(8.20058408060299,1.29406305600824,0.605326635812744));
#8966=CARTESIAN_POINT('Ctrl Pts',(7.29999999953093,1.32031613471704,0.605285370449856));
#8967=CARTESIAN_POINT('',(9.99999999523418,1.1090098672342,0.7));
#8968=CARTESIAN_POINT('Ctrl Pts',(9.99999999968202,1.20899340489109,0.605457329065633));
#8969=CARTESIAN_POINT('Ctrl Pts',(9.99999999887489,1.20856043137698,0.613368813757176));
#8970=CARTESIAN_POINT('Ctrl Pts',(9.99999852309337,1.20715974444566,0.621187403383205));
#8971=CARTESIAN_POINT('Ctrl Pts',(9.99999786661901,1.20487567413208,0.628752957409046));
#8972=CARTESIAN_POINT('Ctrl Pts',(9.9999975031266,1.20361097553651,0.63294203403));
#8973=CARTESIAN_POINT('Ctrl Pts',(9.99999733971606,1.20207445367248,0.63705356322819));
#8974=CARTESIAN_POINT('Ctrl Pts',(9.99999742766416,1.20027388348257,0.64105842070465));
#8975=CARTESIAN_POINT('Ctrl Pts',(9.9999975865154,1.19702170610966,0.6482919664668));
#8976=CARTESIAN_POINT('Ctrl Pts',(9.99999868569093,1.19294650045069,0.655099368158521));
#8977=CARTESIAN_POINT('Ctrl Pts',(9.9999991134218,1.18811276085989,0.661317774786376));
#8978=CARTESIAN_POINT('Ctrl Pts',(9.99999919410111,1.18720101282252,0.662490701033652));
#8979=CARTESIAN_POINT('Ctrl Pts',(9.99999924414009,1.18626214680169,0.663642601192937));
#8980=CARTESIAN_POINT('Ctrl Pts',(9.99999924372355,1.18529642131707,0.664772262763739));
#8981=CARTESIAN_POINT('Ctrl Pts',(9.99999924291654,1.18342543943696,0.666960851926287));
#8982=CARTESIAN_POINT('Ctrl Pts',(9.99999905429896,1.18145367213587,0.669066014649603));
#8983=CARTESIAN_POINT('Ctrl Pts',(9.99999879621773,1.17938809187152,0.671084194359814));
#8984=CARTESIAN_POINT('Ctrl Pts',(9.99999808597787,1.17370361260899,0.676638227242868));
#8985=CARTESIAN_POINT('Ctrl Pts',(9.9999969699445,1.16737553754052,0.681473799108647));
#8986=CARTESIAN_POINT('Ctrl Pts',(9.99999660204079,1.16056788011185,0.685537070165577));
#8987=CARTESIAN_POINT('Ctrl Pts',(9.99999636768906,1.15623145667386,0.688125341392612));
#8988=CARTESIAN_POINT('Ctrl Pts',(9.99999638726733,1.15169947441128,0.690399565850749));
#8989=CARTESIAN_POINT('Ctrl Pts',(9.99999666360534,1.14700857532255,0.692336497939236));
#8990=CARTESIAN_POINT('Ctrl Pts',(9.99999709503399,1.13968497812548,0.695360504669253));
#8991=CARTESIAN_POINT('Ctrl Pts',(9.99999815490668,1.13205884654683,0.697530003145419));
#8992=CARTESIAN_POINT('Ctrl Pts',(9.99999900983214,1.12427739544825,0.698775573347137));
#8993=CARTESIAN_POINT('Ctrl Pts',(9.99999956314479,1.11924119569193,0.699581713521624));
#8994=CARTESIAN_POINT('Ctrl Pts',(10.,1.11413933950174,0.7));
#8995=CARTESIAN_POINT('Ctrl Pts',(10.,1.10900986674273,0.7));
#8996=CARTESIAN_POINT('Ctrl Pts',(8.26514054272776,1.18768929227839,0.7));
#8997=CARTESIAN_POINT('Ctrl Pts',(8.84359655063997,1.16547286645366,0.7));
#8998=CARTESIAN_POINT('Ctrl Pts',(9.42188471826001,1.13881853081542,0.7));
#8999=CARTESIAN_POINT('Ctrl Pts',(9.99999999522154,1.10900986698912,0.7));
#9000=CARTESIAN_POINT('Origin',(5.4,-8.11656130105013E-18,0.7));
#9001=CARTESIAN_POINT('',(7.3,-1.22041345053557,0.7));
#9002=CARTESIAN_POINT('Ctrl Pts',(7.94916654049851,-1.19937499624794,0.7));
#9003=CARTESIAN_POINT('Ctrl Pts',(7.73280095382446,-1.20706364505454,0.7));
#9004=CARTESIAN_POINT('Ctrl Pts',(7.51641201888728,-1.21409884616656,0.7));
#9005=CARTESIAN_POINT('Ctrl Pts',(7.29999999989085,-1.22041345054982,0.7));
#9006=CARTESIAN_POINT('',(7.3,-0.712777777777778,0.7));
#9007=CARTESIAN_POINT('',(10.,-1.10900986674244,0.7));
#9008=CARTESIAN_POINT('',(10.,0.653773457742722,0.7));
#9009=CARTESIAN_POINT('Ctrl Pts',(10.,-1.10900986674273,0.7));
#9010=CARTESIAN_POINT('Ctrl Pts',(9.42188472144661,-1.13881853066854,0.7));
#9011=CARTESIAN_POINT('Ctrl Pts',(8.84359655223373,-1.16547286639245,0.7));
#9012=CARTESIAN_POINT('Ctrl Pts',(8.26514054272776,-1.18768929227839,0.7));
#9013=CARTESIAN_POINT('',(7.95,-1.,0.7));
#9014=CARTESIAN_POINT('Origin',(8.1,-1.,0.7));
#9015=CARTESIAN_POINT('',(7.95,1.,0.7));
#9016=CARTESIAN_POINT('Origin',(8.1,1.,0.7));
#9017=CARTESIAN_POINT('',(8.4,-4.89858719658942E-17,0.7));
#9018=CARTESIAN_POINT('Origin',(8.8,0.,0.7));
#9019=CARTESIAN_POINT('Origin',(8.1,-1.,0.8));
#9020=CARTESIAN_POINT('',(7.95,-1.,0.9));
#9021=CARTESIAN_POINT('Origin',(8.1,-1.,0.9));
#9022=CARTESIAN_POINT('',(7.95,-1.,0.8));
#9023=CARTESIAN_POINT('Origin',(2.7,-1.,0.8));
#9024=CARTESIAN_POINT('',(2.55,-1.,0.9));
#9025=CARTESIAN_POINT('Origin',(2.7,-1.,0.9));
#9026=CARTESIAN_POINT('',(2.55,-1.,0.7));
#9027=CARTESIAN_POINT('',(2.55,-1.,0.8));
#9028=CARTESIAN_POINT('Origin',(2.7,-1.,0.7));
#9029=CARTESIAN_POINT('Origin',(2.7,1.,0.8));
#9030=CARTESIAN_POINT('',(2.55,1.,0.9));
#9031=CARTESIAN_POINT('Origin',(2.7,1.,0.9));
#9032=CARTESIAN_POINT('',(2.55,1.,0.7));
#9033=CARTESIAN_POINT('',(2.55,1.,0.8));
#9034=CARTESIAN_POINT('Origin',(2.7,1.,0.7));
#9035=CARTESIAN_POINT('Origin',(8.1,1.,0.8));
#9036=CARTESIAN_POINT('',(7.95,1.,0.9));
#9037=CARTESIAN_POINT('Origin',(8.1,1.,0.9));
#9038=CARTESIAN_POINT('',(7.95,1.,0.8));
#9039=CARTESIAN_POINT('Origin',(2.,0.,0.75));
#9040=CARTESIAN_POINT('',(1.7,3.67394039744206E-17,0.9));
#9041=CARTESIAN_POINT('Origin',(2.,0.,0.9));
#9042=CARTESIAN_POINT('',(1.7,3.67394039744206E-17,0.6));
#9043=CARTESIAN_POINT('',(1.7,3.67394039744206E-17,0.75));
#9044=CARTESIAN_POINT('Origin',(2.,0.,0.6));
#9045=CARTESIAN_POINT('Origin',(2.,0.,0.6));
#9046=CARTESIAN_POINT('',(1.83,-2.0818995585505E-17,0.6));
#9047=CARTESIAN_POINT('Origin',(2.,0.,0.6));
#9048=CARTESIAN_POINT('Origin',(8.8,0.,0.75));
#9049=CARTESIAN_POINT('',(8.5,3.67394039744206E-17,0.9));
#9050=CARTESIAN_POINT('Origin',(8.8,0.,0.9));
#9051=CARTESIAN_POINT('',(8.5,3.67394039744206E-17,0.6));
#9052=CARTESIAN_POINT('',(8.5,3.67394039744206E-17,0.75));
#9053=CARTESIAN_POINT('Origin',(8.8,0.,0.6));
#9054=CARTESIAN_POINT('Origin',(8.8,0.,0.6));
#9055=CARTESIAN_POINT('',(8.63,-2.0818995585505E-17,0.6));
#9056=CARTESIAN_POINT('Origin',(8.8,0.,0.6));
#9057=CARTESIAN_POINT('Origin',(2.,0.,0.45));
#9058=CARTESIAN_POINT('',(1.83,-2.0818995585505E-17,0.32));
#9059=CARTESIAN_POINT('',(1.83,2.0818995585505E-17,0.45));
#9060=CARTESIAN_POINT('Origin',(2.,0.,0.32));
#9061=CARTESIAN_POINT('Origin',(8.8,0.,0.45));
#9062=CARTESIAN_POINT('',(8.63,-2.0818995585505E-17,0.32));
#9063=CARTESIAN_POINT('',(8.63,2.0818995585505E-17,0.45));
#9064=CARTESIAN_POINT('Origin',(8.8,0.,0.32));
#9065=CARTESIAN_POINT('Origin',(10.,-0.62,0.32));
#9066=CARTESIAN_POINT('',(0.200274469199584,-0.62,0.));
#9067=CARTESIAN_POINT('',(0.217044958570157,-0.62,0.32));
#9068=CARTESIAN_POINT('',(0.221783445591644,-0.62,0.410415718550007));
#9069=CARTESIAN_POINT('',(0.,-0.62,0.));
#9070=CARTESIAN_POINT('',(7.7,-0.62,0.));
#9071=CARTESIAN_POINT('',(0.0167704893705732,-0.62,0.32));
#9072=CARTESIAN_POINT('',(0.0220575386407278,-0.62,0.420882909798596));
#9073=CARTESIAN_POINT('',(-0.1,-0.62,0.32));
#9074=CARTESIAN_POINT('Origin',(10.,-0.62,0.32));
#9075=CARTESIAN_POINT('',(0.9,-0.62,0.32));
#9076=CARTESIAN_POINT('',(0.9,-0.62,0.));
#9077=CARTESIAN_POINT('',(0.9,-0.62,0.16));
#9078=CARTESIAN_POINT('',(1.1,-0.62,0.32));
#9079=CARTESIAN_POINT('',(-0.1,-0.62,0.32));
#9080=CARTESIAN_POINT('',(1.1,-0.62,0.));
#9081=CARTESIAN_POINT('',(1.1,-0.62,0.16));
#9082=CARTESIAN_POINT('',(7.7,-0.62,0.));
#9083=CARTESIAN_POINT('Origin',(10.,-0.62,0.32));
#9084=CARTESIAN_POINT('',(3.5,-0.62,0.32));
#9085=CARTESIAN_POINT('',(3.5,-0.62,0.));
#9086=CARTESIAN_POINT('',(3.5,-0.62,0.16));
#9087=CARTESIAN_POINT('',(3.7,-0.62,0.32));
#9088=CARTESIAN_POINT('',(-0.1,-0.62,0.32));
#9089=CARTESIAN_POINT('',(3.7,-0.62,0.));
#9090=CARTESIAN_POINT('',(3.7,-0.62,0.16));
#9091=CARTESIAN_POINT('',(7.7,-0.62,0.));
#9092=CARTESIAN_POINT('Origin',(10.,-0.62,0.32));
#9093=CARTESIAN_POINT('',(7.1,-0.62,0.32));
#9094=CARTESIAN_POINT('',(7.1,-0.62,0.));
#9095=CARTESIAN_POINT('',(7.1,-0.62,0.16));
#9096=CARTESIAN_POINT('',(7.3,-0.62,0.32));
#9097=CARTESIAN_POINT('',(-0.1,-0.62,0.32));
#9098=CARTESIAN_POINT('',(7.3,-0.62,0.));
#9099=CARTESIAN_POINT('',(7.3,-0.62,0.16));
#9100=CARTESIAN_POINT('',(7.7,-0.62,0.));
#9101=CARTESIAN_POINT('Origin',(-0.0999999999999996,0.62,0.32));
#9102=CARTESIAN_POINT('',(0.217044958570158,0.62,0.32));
#9103=CARTESIAN_POINT('',(0.200274469199584,0.62,0.));
#9104=CARTESIAN_POINT('',(0.207951231396534,0.62,0.146481348799182));
#9105=CARTESIAN_POINT('',(0.0167704893705736,0.62,0.32));
#9106=CARTESIAN_POINT('',(10.,0.62,0.32));
#9107=CARTESIAN_POINT('',(0.,0.62,0.));
#9108=CARTESIAN_POINT('',(0.00822532444561912,0.62,0.156948540047771));
#9109=CARTESIAN_POINT('',(2.65,0.62,0.));
#9110=CARTESIAN_POINT('Origin',(-0.0999999999999996,0.62,0.32));
#9111=CARTESIAN_POINT('',(0.9,0.62,0.));
#9112=CARTESIAN_POINT('',(0.9,0.62,0.32));
#9113=CARTESIAN_POINT('',(0.9,0.62,0.16));
#9114=CARTESIAN_POINT('',(1.1,0.62,0.));
#9115=CARTESIAN_POINT('',(2.65,0.62,0.));
#9116=CARTESIAN_POINT('',(1.1,0.62,0.32));
#9117=CARTESIAN_POINT('',(1.1,0.62,0.16));
#9118=CARTESIAN_POINT('',(10.,0.62,0.32));
#9119=CARTESIAN_POINT('Origin',(-0.0999999999999996,0.62,0.32));
#9120=CARTESIAN_POINT('',(3.5,0.62,0.));
#9121=CARTESIAN_POINT('',(3.5,0.62,0.32));
#9122=CARTESIAN_POINT('',(3.5,0.62,0.16));
#9123=CARTESIAN_POINT('',(3.7,0.62,0.));
#9124=CARTESIAN_POINT('',(2.65,0.62,0.));
#9125=CARTESIAN_POINT('',(3.7,0.62,0.32));
#9126=CARTESIAN_POINT('',(3.7,0.62,0.16));
#9127=CARTESIAN_POINT('',(10.,0.62,0.32));
#9128=CARTESIAN_POINT('Origin',(4.95,0.,0.32));
#9129=CARTESIAN_POINT('',(1.6,-4.89858719658941E-17,0.32));
#9130=CARTESIAN_POINT('Origin',(2.,0.,0.32));
#9131=CARTESIAN_POINT('Origin',(4.95,0.,0.32));
#9132=CARTESIAN_POINT('',(8.4,-4.89858719658942E-17,0.32));
#9133=CARTESIAN_POINT('Origin',(8.8,0.,0.32));
#9134=CARTESIAN_POINT('Origin',(4.95,0.,0.32));
#9135=CARTESIAN_POINT('',(0.217044958570157,-0.7,0.32));
#9136=CARTESIAN_POINT('',(0.0167704893705731,-0.7,0.32));
#9137=CARTESIAN_POINT('Origin',(4.95,0.,0.32));
#9138=CARTESIAN_POINT('',(0.9,0.671641708581009,0.32));
#9139=CARTESIAN_POINT('',(1.1,-0.671641708581009,0.32));
#9140=CARTESIAN_POINT('Origin',(4.95,0.,0.32));
#9141=CARTESIAN_POINT('',(3.5,0.723888888888889,0.32));
#9142=CARTESIAN_POINT('',(3.7,-0.723888888888889,0.32));
#9143=CARTESIAN_POINT('Origin',(4.95,0.,0.32));
#9144=CARTESIAN_POINT('',(7.1,0.62,0.32));
#9145=CARTESIAN_POINT('',(7.1,0.712777777777778,0.32));
#9146=CARTESIAN_POINT('',(7.3,0.62,0.32));
#9147=CARTESIAN_POINT('',(10.,0.62,0.32));
#9148=CARTESIAN_POINT('',(7.3,-0.712777777777778,0.32));
#9149=CARTESIAN_POINT('Origin',(-0.0999999999999996,0.62,0.32));
#9150=CARTESIAN_POINT('',(7.1,0.62,0.));
#9151=CARTESIAN_POINT('',(7.1,0.62,0.16));
#9152=CARTESIAN_POINT('',(7.3,0.62,0.));
#9153=CARTESIAN_POINT('',(2.65,0.62,0.));
#9154=CARTESIAN_POINT('',(7.3,0.62,0.16));
#9155=CARTESIAN_POINT('Origin',(10.,1.30754691548544,0.));
#9156=CARTESIAN_POINT('',(10.,1.24211782565704,0.));
#9157=CARTESIAN_POINT('',(10.,-1.24211782565704,0.));
#9158=CARTESIAN_POINT('',(10.,1.30754691548544,0.));
#9159=CARTESIAN_POINT('',(10.,-1.20899340483173,0.605457329065657));
#9160=CARTESIAN_POINT('Ctrl Pts',(10.,-1.20899340483173,0.605457329065657));
#9161=CARTESIAN_POINT('Ctrl Pts',(10.,-1.21451837038612,0.504502771559899));
#9162=CARTESIAN_POINT('Ctrl Pts',(10.,-1.22004249263249,0.403547366186347));
#9163=CARTESIAN_POINT('Ctrl Pts',(10.,-1.23108392958594,0.201728789021226));
#9164=CARTESIAN_POINT('Ctrl Pts',(10.,-1.23660133320922,0.100864020914724));
#9165=CARTESIAN_POINT('Ctrl Pts',(10.,-1.24211782565704,0.));
#9166=CARTESIAN_POINT('Ctrl Pts',(10.,-1.10900986674273,0.7));
#9167=CARTESIAN_POINT('Ctrl Pts',(10.,-1.11692706738765,0.7));
#9168=CARTESIAN_POINT('Ctrl Pts',(9.99999896020971,-1.12478097169818,0.699006158364426));
#9169=CARTESIAN_POINT('Ctrl Pts',(9.99999805494427,-1.13243115645175,0.697118998397561));
#9170=CARTESIAN_POINT('Ctrl Pts',(9.99999754769332,-1.13671781459207,0.696061558623929));
#9171=CARTESIAN_POINT('Ctrl Pts',(9.99999708556116,-1.14094056283945,0.694722610426682));
#9172=CARTESIAN_POINT('Ctrl Pts',(9.99999679002998,-1.14507302265453,0.693112977943955));
#9173=CARTESIAN_POINT('Ctrl Pts',(9.99999625879002,-1.15250143622127,0.690219540062595));
#9174=CARTESIAN_POINT('Ctrl Pts',(9.999996365957,-1.15955821040664,0.686485807665162));
#9175=CARTESIAN_POINT('Ctrl Pts',(9.99999703387985,-1.16609707610076,0.681992895329386));
#9176=CARTESIAN_POINT('Ctrl Pts',(9.99999740034986,-1.16968476316425,0.679527763880215));
#9177=CARTESIAN_POINT('Ctrl Pts',(9.99999792190556,-1.17311627083768,0.676833210412541));
#9178=CARTESIAN_POINT('Ctrl Pts',(9.99999838578331,-1.17636354905877,0.673917165661822));
#9179=CARTESIAN_POINT('Ctrl Pts',(9.99999884023993,-1.17954487655573,0.671060344436104));
#9180=CARTESIAN_POINT('Ctrl Pts',(9.99999924462882,-1.18253006594632,0.668008218820746));
#9181=CARTESIAN_POINT('Ctrl Pts',(9.99999924442301,-1.185296421281,0.664772262763763));
#9182=CARTESIAN_POINT('Ctrl Pts',(9.99999924404215,-1.19041578560695,0.658783864313737));
#9183=CARTESIAN_POINT('Ctrl Pts',(9.99999800949836,-1.19478865237554,0.652167294255586));
#9184=CARTESIAN_POINT('Ctrl Pts',(9.99999759228052,-1.19835462180986,0.645087621913151));
#9185=CARTESIAN_POINT('Ctrl Pts',(9.99999755030119,-1.19871341999785,0.644375284453517));
#9186=CARTESIAN_POINT('Ctrl Pts',(9.9999975145836,-1.19906401030029,0.643658239626438));
#9187=CARTESIAN_POINT('Ctrl Pts',(9.99999748581823,-1.19940630408966,0.642936645100882));
#9188=CARTESIAN_POINT('Ctrl Pts',(9.99999720003888,-1.20280693749908,0.635767720253638));
#9189=CARTESIAN_POINT('Ctrl Pts',(9.9999978299417,-1.20535324884233,0.628234501710241));
#9190=CARTESIAN_POINT('Ctrl Pts',(9.99999874867777,-1.20699142055415,0.62050509267719));
#9191=CARTESIAN_POINT('Ctrl Pts',(9.99999933690345,-1.20804026874419,0.615556297251186));
#9192=CARTESIAN_POINT('Ctrl Pts',(9.99999999916487,-1.20871598809812,0.61052641213707));
#9193=CARTESIAN_POINT('Ctrl Pts',(9.99999999968202,-1.20899340489109,0.605457329065633));
#9194=CARTESIAN_POINT('Ctrl Pts',(10.,1.24211782565704,0.));
#9195=CARTESIAN_POINT('Ctrl Pts',(10.,1.23660053043673,0.100878698875723));
#9196=CARTESIAN_POINT('Ctrl Pts',(10.,1.23108232376984,0.201758145268796));
#9197=CARTESIAN_POINT('Ctrl Pts',(10.,1.22004088630648,0.403576722396156));
#9198=CARTESIAN_POINT('Ctrl Pts',(10.,1.2145175671044,0.504517449470448));
#9199=CARTESIAN_POINT('Ctrl Pts',(10.,1.20899340483173,0.605457329065657));
#9200=CARTESIAN_POINT('Origin',(7.3,-1.42555555555556,0.));
#9201=CARTESIAN_POINT('',(7.3,1.35236351479115,0.));
#9202=CARTESIAN_POINT('',(7.3,-1.42555555555556,0.));
#9203=CARTESIAN_POINT('Ctrl Pts',(7.29999999953133,1.3203161347307,0.605285370449834));
#9204=CARTESIAN_POINT('Ctrl Pts',(7.29999999953133,1.32565322760551,0.504490726585133));
#9205=CARTESIAN_POINT('Ctrl Pts',(7.3,1.33099015509697,0.403695123734478));
#9206=CARTESIAN_POINT('Ctrl Pts',(7.3,1.34167258064689,0.201933969199042));
#9207=CARTESIAN_POINT('Ctrl Pts',(7.3,1.34701817868136,0.100966514951419));
#9208=CARTESIAN_POINT('Ctrl Pts',(7.3,1.35236351479115,0.));
#9209=CARTESIAN_POINT('',(7.29999999953133,-1.3203161347307,0.605285370449834));
#9210=CARTESIAN_POINT('Ctrl Pts',(7.3,-1.32031613470337,0.605285370449877));
#9211=CARTESIAN_POINT('Ctrl Pts',(7.3,-1.31989712778929,0.61319860217968));
#9212=CARTESIAN_POINT('Ctrl Pts',(7.29999916171872,-1.31851071739963,0.621020829077898));
#9213=CARTESIAN_POINT('Ctrl Pts',(7.29999878808195,-1.31624092632926,0.628591660945423));
#9214=CARTESIAN_POINT('Ctrl Pts',(7.29999857947278,-1.31497365483497,0.632818613610392));
#9215=CARTESIAN_POINT('Ctrl Pts',(7.29999848639856,-1.31343001415,0.636967235874856));
#9216=CARTESIAN_POINT('Ctrl Pts',(7.29999853830689,-1.31161789606625,0.641007613679984));
#9217=CARTESIAN_POINT('Ctrl Pts',(7.29999863125487,-1.30837308502546,0.648242386418365));
#9218=CARTESIAN_POINT('Ctrl Pts',(7.29999925734287,-1.30430566789097,0.655052076019481));
#9219=CARTESIAN_POINT('Ctrl Pts',(7.29999949821933,-1.29947941328181,0.661273460789274));
#9220=CARTESIAN_POINT('Ctrl Pts',(7.29999954322,-1.29857776968225,0.662435743389828));
#9221=CARTESIAN_POINT('Ctrl Pts',(7.29999957102613,-1.29764951297213,0.663577423078133));
#9222=CARTESIAN_POINT('Ctrl Pts',(7.2999995707084,-1.29669488998092,0.664697318929248));
#9223=CARTESIAN_POINT('Ctrl Pts',(7.29999957007561,-1.29479368240016,0.666927680549918));
#9224=CARTESIAN_POINT('Ctrl Pts',(7.29999945886743,-1.29278792931167,0.669071688571899));
#9225=CARTESIAN_POINT('Ctrl Pts',(7.29999930790078,-1.2906849717248,0.671125563583336));
#9226=CARTESIAN_POINT('Ctrl Pts',(7.29999889984047,-1.28500071247856,0.676677153447665));
#9227=CARTESIAN_POINT('Ctrl Pts',(7.29999826931494,-1.27867319504519,0.681510485910933));
#9228=CARTESIAN_POINT('Ctrl Pts',(7.29999806345125,-1.27186607945067,0.685571085769401));
#9229=CARTESIAN_POINT('Ctrl Pts',(7.29999793266427,-1.26754145993833,0.688150820039508));
#9230=CARTESIAN_POINT('Ctrl Pts',(7.29999794545359,-1.26302231037287,0.690417984675215));
#9231=CARTESIAN_POINT('Ctrl Pts',(7.29999810371711,-1.25834494218995,0.69234933099425));
#9232=CARTESIAN_POINT('Ctrl Pts',(7.29999835129001,-1.25102809722258,0.695370551698293));
#9233=CARTESIAN_POINT('Ctrl Pts',(7.29999895574222,-1.24340909242398,0.6975375590939));
#9234=CARTESIAN_POINT('Ctrl Pts',(7.29999944081525,-1.2356348173965,0.698780605629559));
#9235=CARTESIAN_POINT('Ctrl Pts',(7.29999975409932,-1.23061380764338,0.699583426311495));
#9236=CARTESIAN_POINT('Ctrl Pts',(7.30000000047446,-1.22552743956586,0.699999999832051));
#9237=CARTESIAN_POINT('Ctrl Pts',(7.29999999989087,-1.22041345054982,0.7));
#9238=CARTESIAN_POINT('',(7.3,-1.35236351479115,0.));
#9239=CARTESIAN_POINT('Ctrl Pts',(7.3,-1.35236351479115,0.));
#9240=CARTESIAN_POINT('Ctrl Pts',(7.3,-1.34701814920095,0.100967071798286));
#9241=CARTESIAN_POINT('Ctrl Pts',(7.3,-1.34167252169398,0.201935082699409));
#9242=CARTESIAN_POINT('Ctrl Pts',(7.3,-1.33099009614589,0.403696237111114));
#9243=CARTESIAN_POINT('Ctrl Pts',(7.29999999953133,-1.32565319812959,0.504491283257837));
#9244=CARTESIAN_POINT('Ctrl Pts',(7.29999999953133,-1.3203161347307,0.605285370449834));
#9245=CARTESIAN_POINT('',(7.3,-1.42555555555556,0.));
#9246=CARTESIAN_POINT('Origin',(3.7,-1.44777777777778,0.));
#9247=CARTESIAN_POINT('',(3.7,1.37924639543935,0.));
#9248=CARTESIAN_POINT('',(3.7,-1.44777777777778,0.));
#9249=CARTESIAN_POINT('',(3.7,1.34735368793805,0.605261457205193));
#9250=CARTESIAN_POINT('Ctrl Pts',(3.7,1.34735368793805,0.605261457205193));
#9251=CARTESIAN_POINT('Ctrl Pts',(3.7,1.35266395147774,0.504488703431434));
#9252=CARTESIAN_POINT('Ctrl Pts',(3.7,1.35797406404029,0.40371594170176));
#9253=CARTESIAN_POINT('Ctrl Pts',(3.7,1.36860496587027,0.201962122597264));
#9254=CARTESIAN_POINT('Ctrl Pts',(3.7,1.37392575452088,0.100981065191366));
#9255=CARTESIAN_POINT('Ctrl Pts',(3.7,1.37924639543935,0.));
#9256=CARTESIAN_POINT('',(3.7,1.24747724070879,0.7));
#9257=CARTESIAN_POINT('Ctrl Pts',(3.7,1.24747724070879,0.7));
#9258=CARTESIAN_POINT('Ctrl Pts',(3.7,1.25538532734776,0.7));
#9259=CARTESIAN_POINT('Ctrl Pts',(3.70000034866643,1.26322972530331,0.699006048248363));
#9260=CARTESIAN_POINT('Ctrl Pts',(3.70000065268588,1.27087026624727,0.697119044026295));
#9261=CARTESIAN_POINT('Ctrl Pts',(3.7000008238479,1.27517186762995,0.696056666371322));
#9262=CARTESIAN_POINT('Ctrl Pts',(3.70000097972585,1.27940891103121,0.694710185093394));
#9263=CARTESIAN_POINT('Ctrl Pts',(3.70000107833511,1.28355469746902,0.693090631030141));
#9264=CARTESIAN_POINT('Ctrl Pts',(3.70000125487464,1.29097687270382,0.690191153635441));
#9265=CARTESIAN_POINT('Ctrl Pts',(3.7000012145424,1.29802606517866,0.686451118058958));
#9266=CARTESIAN_POINT('Ctrl Pts',(3.70000098691147,1.3045562506385,0.681952404110064));
#9267=CARTESIAN_POINT('Ctrl Pts',(3.70000086156653,1.30815209635338,0.679475187900035));
#9268=CARTESIAN_POINT('Ctrl Pts',(3.70000068390876,1.31159030769532,0.676767042898431));
#9269=CARTESIAN_POINT('Ctrl Pts',(3.70000052608992,1.31484259178137,0.673836088143417));
#9270=CARTESIAN_POINT('Ctrl Pts',(3.70000037216713,1.31801458722906,0.670977489418868));
#9271=CARTESIAN_POINT('Ctrl Pts',(3.70000023558528,1.32099045552882,0.667924239810466));
#9272=CARTESIAN_POINT('Ctrl Pts',(3.70000023595245,1.32374763345498,0.664687876924229));
#9273=CARTESIAN_POINT('Ctrl Pts',(3.70000023663259,1.32885491153898,0.658692977181302));
#9274=CARTESIAN_POINT('Ctrl Pts',(3.70000065621025,1.33321474659758,0.652071180203097));
#9275=CARTESIAN_POINT('Ctrl Pts',(3.70000080093706,1.33676785491319,0.644988218508662));
#9276=CARTESIAN_POINT('Ctrl Pts',(3.70000081573428,1.33713113341147,0.644264039153811));
#9277=CARTESIAN_POINT('Ctrl Pts',(3.70000082835625,1.33748593861467,0.643535019157411));
#9278=CARTESIAN_POINT('Ctrl Pts',(3.70000083855542,1.33783217873901,0.642801324492746));
#9279=CARTESIAN_POINT('Ctrl Pts',(3.70000093832019,1.34121897990539,0.63562457699476));
#9280=CARTESIAN_POINT('Ctrl Pts',(3.70000072997693,1.34375116782692,0.628085030530103));
#9281=CARTESIAN_POINT('Ctrl Pts',(3.70000042189378,1.34537558692779,0.6203512574804));
#9282=CARTESIAN_POINT('Ctrl Pts',(3.70000022417294,1.3464181026242,0.615387895628485));
#9283=CARTESIAN_POINT('Ctrl Pts',(3.70000000036652,1.34708586836718,0.6103438638189));
#9284=CARTESIAN_POINT('Ctrl Pts',(3.69999999992214,1.34735368792773,0.6052614572053));
#9285=CARTESIAN_POINT('',(3.7,-1.24747724070944,0.7));
#9286=CARTESIAN_POINT('',(3.7,-0.723888888888889,0.7));
#9287=CARTESIAN_POINT('',(3.7,-1.34735368793805,0.605261457205193));
#9288=CARTESIAN_POINT('Ctrl Pts',(3.69999999992215,-1.34735368792773,0.6052614572053));
#9289=CARTESIAN_POINT('Ctrl Pts',(3.70000000061408,-1.34693666923469,0.613175212866596));
#9290=CARTESIAN_POINT('Ctrl Pts',(3.70000049671034,-1.34555248374866,0.620998392122869));
#9291=CARTESIAN_POINT('Ctrl Pts',(3.70000071566022,-1.34328499565267,0.628570462735333));
#9292=CARTESIAN_POINT('Ctrl Pts',(3.70000083807517,-1.34201724238155,0.632804009674372));
#9293=CARTESIAN_POINT('Ctrl Pts',(3.7000008913247,-1.34047237297042,0.63695909738719));
#9294=CARTESIAN_POINT('Ctrl Pts',(3.70000085837557,-1.33865827982058,0.641005656934072));
#9295=CARTESIAN_POINT('Ctrl Pts',(3.7000007994669,-1.33541492172585,0.648240369034365));
#9296=CARTESIAN_POINT('Ctrl Pts',(3.70000042420685,-1.33134915897915,0.655050234746405));
#9297=CARTESIAN_POINT('Ctrl Pts',(3.70000027984635,-1.32652447879733,0.661271863919233));
#9298=CARTESIAN_POINT('Ctrl Pts',(3.70000025294096,-1.32562527203035,0.662431429080655));
#9299=CARTESIAN_POINT('Ctrl Pts',(3.7000002362737,-1.32469957579387,0.663570491348455));
#9300=CARTESIAN_POINT('Ctrl Pts',(3.70000023630138,-1.32374763346102,0.664687876924223));
#9301=CARTESIAN_POINT('Ctrl Pts',(3.70000023635686,-1.32184039796576,0.666926581264246));
#9302=CARTESIAN_POINT('Ctrl Pts',(3.70000030283857,-1.31982784222224,0.669078323867587));
#9303=CARTESIAN_POINT('Ctrl Pts',(3.70000039320883,-1.31771738411303,0.671139279696989));
#9304=CARTESIAN_POINT('Ctrl Pts',(3.70000063660146,-1.3120333248939,0.676690015307994));
#9305=CARTESIAN_POINT('Ctrl Pts',(3.7000010126336,-1.30570602994251,0.681522474044465));
#9306=CARTESIAN_POINT('Ctrl Pts',(3.70000113724274,-1.29889910811053,0.685582059356066));
#9307=CARTESIAN_POINT('Ctrl Pts',(3.70000121634872,-1.29457784995583,0.688159217808216));
#9308=CARTESIAN_POINT('Ctrl Pts',(3.70000121058612,-1.2900623422215,0.690424215862126));
#9309=CARTESIAN_POINT('Ctrl Pts',(3.70000111831253,-1.28538881676413,0.692353818784707));
#9310=CARTESIAN_POINT('Ctrl Pts',(3.70000097388434,-1.27807373536961,0.695374066040565));
#9311=CARTESIAN_POINT('Ctrl Pts',(3.70000061691996,-1.27045659963863,0.697540160564298));
#9312=CARTESIAN_POINT('Ctrl Pts',(3.7000003304055,-1.26268427129293,0.698782316368755));
#9313=CARTESIAN_POINT('Ctrl Pts',(3.70000014548661,-1.25766794365683,0.699584014420239));
#9314=CARTESIAN_POINT('Ctrl Pts',(3.7,-1.25258637988459,0.7));
#9315=CARTESIAN_POINT('Ctrl Pts',(3.7,-1.24747724070879,0.7));
#9316=CARTESIAN_POINT('',(3.7,-1.37924639543935,0.));
#9317=CARTESIAN_POINT('Ctrl Pts',(3.7,-1.37924639543935,0.));
#9318=CARTESIAN_POINT('Ctrl Pts',(3.7,-1.37392574223662,0.100981298335747));
#9319=CARTESIAN_POINT('Ctrl Pts',(3.7,-1.36860494130098,0.201962588887634));
#9320=CARTESIAN_POINT('Ctrl Pts',(3.7,-1.35797403946962,0.403716407992068));
#9321=CARTESIAN_POINT('Ctrl Pts',(3.7,-1.3526639391921,0.504488936575732));
#9322=CARTESIAN_POINT('Ctrl Pts',(3.7,-1.34735368793805,0.605261457205193));
#9323=CARTESIAN_POINT('',(3.7,-1.44777777777778,0.));
#9324=CARTESIAN_POINT('Origin',(1.1,-1.34328341716202,0.));
#9325=CARTESIAN_POINT('',(1.1,1.27885335043294,0.));
#9326=CARTESIAN_POINT('',(1.1,-1.34328341716202,0.));
#9327=CARTESIAN_POINT('Ctrl Pts',(1.1,1.24553911298206,0.605485603995113));
#9328=CARTESIAN_POINT('Ctrl Pts',(1.1,1.25109559382646,0.504544105903265));
#9329=CARTESIAN_POINT('Ctrl Pts',(1.1,1.25665083308595,0.403601248768354));
#9330=CARTESIAN_POINT('Ctrl Pts',(1.1,1.26775551906787,0.201773573764085));
#9331=CARTESIAN_POINT('Ctrl Pts',(1.1,1.2733051088238,0.100886182270816));
#9332=CARTESIAN_POINT('Ctrl Pts',(1.1,1.27885335043294,0.));
#9333=CARTESIAN_POINT('',(1.1,-1.14549341399195,0.7));
#9334=CARTESIAN_POINT('',(1.1,-0.671641708581009,0.7));
#9335=CARTESIAN_POINT('',(1.1,-1.24553911298206,0.605485603995113));
#9336=CARTESIAN_POINT('Ctrl Pts',(1.09999999916631,-1.24553911263843,0.605485603997431));
#9337=CARTESIAN_POINT('Ctrl Pts',(1.10000000220634,-1.24510362317222,0.61339691285734));
#9338=CARTESIAN_POINT('Ctrl Pts',(1.10000177015643,-1.24370036622144,0.621215229994996));
#9339=CARTESIAN_POINT('Ctrl Pts',(1.10000252895322,-1.24141353486351,0.628780213666851));
#9340=CARTESIAN_POINT('Ctrl Pts',(1.10000294802756,-1.24015054543059,0.632958263090869));
#9341=CARTESIAN_POINT('Ctrl Pts',(1.10000312162076,-1.23861706177488,0.637059070655947));
#9342=CARTESIAN_POINT('Ctrl Pts',(1.10000299297862,-1.23682078380192,0.641053713130525));
#9343=CARTESIAN_POINT('Ctrl Pts',(1.10000275999609,-1.23356756237267,0.64828837095969));
#9344=CARTESIAN_POINT('Ctrl Pts',(1.10000138715103,-1.22949085733774,0.655096441442141));
#9345=CARTESIAN_POINT('Ctrl Pts',(1.10000084482056,-1.2246552743941,0.661315040399663));
#9346=CARTESIAN_POINT('Ctrl Pts',(1.10000074196669,-1.22373819809959,0.662494407966206));
#9347=CARTESIAN_POINT('Ctrl Pts',(1.1000006773267,-1.22279369438101,0.663652502541609));
#9348=CARTESIAN_POINT('Ctrl Pts',(1.10000067553493,-1.22182202641035,0.66478809188211));
#9349=CARTESIAN_POINT('Ctrl Pts',(1.10000067210542,-1.219962222636,0.666961646435043));
#9350=CARTESIAN_POINT('Ctrl Pts',(1.10000089707048,-1.21800293160495,0.669052796220007));
#9351=CARTESIAN_POINT('Ctrl Pts',(1.10000120920309,-1.21595100691259,0.671058078730413));
#9352=CARTESIAN_POINT('Ctrl Pts',(1.10000207391986,-1.21026645613745,0.676613414309409));
#9353=CARTESIAN_POINT('Ctrl Pts',(1.1000034579227,-1.20393786500476,0.681450029097565));
#9354=CARTESIAN_POINT('Ctrl Pts',(1.10000394126019,-1.19712964857754,0.685514663758263));
#9355=CARTESIAN_POINT('Ctrl Pts',(1.10000424974863,-1.19278432848208,0.688108902478585));
#9356=CARTESIAN_POINT('Ctrl Pts',(1.10000425197701,-1.18824265871575,0.690387991283085));
#9357=CARTESIAN_POINT('Ctrl Pts',(1.10000394032285,-1.18354156621637,0.692328715646671));
#9358=CARTESIAN_POINT('Ctrl Pts',(1.10000345443802,-1.17621232165581,0.695354404566264));
#9359=CARTESIAN_POINT('Ctrl Pts',(1.10000219938511,-1.16858027633095,0.697525330589554));
#9360=CARTESIAN_POINT('Ctrl Pts',(1.10000118192936,-1.16079305972554,0.698772417158578));
#9361=CARTESIAN_POINT('Ctrl Pts',(1.10000052251962,-1.15574619011492,0.699580649884844));
#9362=CARTESIAN_POINT('Ctrl Pts',(1.1,-1.15063354328712,0.7));
#9363=CARTESIAN_POINT('Ctrl Pts',(1.1,-1.14549341399196,0.7));
#9364=CARTESIAN_POINT('',(1.1,-1.27885335043294,0.));
#9365=CARTESIAN_POINT('Ctrl Pts',(1.1,-1.27885335043294,0.));
#9366=CARTESIAN_POINT('Ctrl Pts',(1.1,-1.27330503870861,0.100887457206881));
#9367=CARTESIAN_POINT('Ctrl Pts',(1.1,-1.26775537880223,0.201776123688554));
#9368=CARTESIAN_POINT('Ctrl Pts',(1.1,-1.25665069275548,0.403603798678134));
#9369=CARTESIAN_POINT('Ctrl Pts',(1.1,-1.25109552364596,0.504545380833391));
#9370=CARTESIAN_POINT('Ctrl Pts',(1.1,-1.24553911298206,0.605485603995113));
#9371=CARTESIAN_POINT('',(1.1,-1.34328341716202,0.));
#9372=CARTESIAN_POINT('Origin',(0.199725906950915,-1.4,-0.0104671912485888));
#9373=CARTESIAN_POINT('',(0.200274469199584,1.12301388185427,1.38777878078145E-17));
#9374=CARTESIAN_POINT('',(0.200274469199585,-0.7,0.));
#9375=CARTESIAN_POINT('',(0.231993417893744,1.09142177001972,0.605233595624295));
#9376=CARTESIAN_POINT('Ctrl Pts',(0.200274469199584,1.12301388185427,-2.97071395261028E-17));
#9377=CARTESIAN_POINT('Ctrl Pts',(0.210847451470635,1.11248294808,0.201744519910852));
#9378=CARTESIAN_POINT('Ctrl Pts',(0.22142043436526,1.101952242875,0.403489051720196));
#9379=CARTESIAN_POINT('Ctrl Pts',(0.231993417893744,1.09142177001972,0.605233595624295));
#9380=CARTESIAN_POINT('',(0.231993417893744,-1.09142177001972,0.605233595624295));
#9381=CARTESIAN_POINT('',(0.231993417893744,-0.7,0.605233595624295));
#9382=CARTESIAN_POINT('',(0.200274469199584,-1.12301388185427,-1.38777878078145E-17));
#9383=CARTESIAN_POINT('Ctrl Pts',(0.231993417893744,-1.09142177001972,0.605233595624295));
#9384=CARTESIAN_POINT('Ctrl Pts',(0.22142043436526,-1.101952242875,0.403489051720196));
#9385=CARTESIAN_POINT('Ctrl Pts',(0.210847451470635,-1.11248294808,0.201744519910852));
#9386=CARTESIAN_POINT('Ctrl Pts',(0.200274469199584,-1.12301388185427,-4.90059381963448E-17));
#9387=CARTESIAN_POINT('',(0.200274469199585,-0.7,0.));
#9388=CARTESIAN_POINT('Origin',(5.4,-1.11022302462516E-16,0.));
#9389=CARTESIAN_POINT('Ctrl Pts',(7.29999999999999,-1.35236351479115,1.04083408558608E-17));
#9390=CARTESIAN_POINT('Ctrl Pts',(8.20044803681595,-1.32637404707459,3.18306896032855E-8));
#9391=CARTESIAN_POINT('Ctrl Pts',(9.10060048441536,-1.28803709316692,1.03188250195688E-8));
#9392=CARTESIAN_POINT('Ctrl Pts',(10.0000000000405,-1.24211782537639,-8.23328475353175E-12));
#9393=CARTESIAN_POINT('Ctrl Pts',(10.0000000000405,1.24211782537639,-8.23320567538283E-12));
#9394=CARTESIAN_POINT('Ctrl Pts',(9.1006004808701,1.28803709334794,1.03184817085883E-8));
#9395=CARTESIAN_POINT('Ctrl Pts',(8.20044803144508,1.32637404722969,3.18291413954212E-8));
#9396=CARTESIAN_POINT('Ctrl Pts',(7.3,1.35236351479115,4.75121773919879E-17));
#9397=CARTESIAN_POINT('',(7.1,1.35793097395724,0.));
#9398=CARTESIAN_POINT('',(7.1,1.42555555555556,0.));
#9399=CARTESIAN_POINT('Ctrl Pts',(7.1000000000396,1.35793097389613,-4.88924676637329E-12));
#9400=CARTESIAN_POINT('Ctrl Pts',(6.53177385320612,1.37316067096195,3.71763852401782E-9));
#9401=CARTESIAN_POINT('Ctrl Pts',(5.96344379069665,1.38333257666104,-3.82408184804385E-8));
#9402=CARTESIAN_POINT('Ctrl Pts',(5.39512359652123,1.38725406840392,-3.97623797275691E-8));
#9403=CARTESIAN_POINT('Ctrl Pts',(4.82973248928002,1.39115534902226,-4.12760989429076E-8));
#9404=CARTESIAN_POINT('Ctrl Pts',(4.26470859812609,1.38886839226708,1.63957607983357E-8));
#9405=CARTESIAN_POINT('Ctrl Pts',(3.70000000036239,1.37924639538501,-6.25376529969227E-12));
#9406=CARTESIAN_POINT('',(3.5,1.37552980833516,0.));
#9407=CARTESIAN_POINT('',(3.5,1.44777777777778,0.));
#9408=CARTESIAN_POINT('Ctrl Pts',(3.50000000097466,1.37552980835479,1.06251812903579E-15));
#9409=CARTESIAN_POINT('Ctrl Pts',(2.69943075695685,1.35940904975719,2.35366119539541E-7));
#9410=CARTESIAN_POINT('Ctrl Pts',(1.89948254587541,1.32827224396921,2.51300192353997E-7));
#9411=CARTESIAN_POINT('Ctrl Pts',(1.10000000028363,1.27885335028943,-5.13283415455519E-11));
#9412=CARTESIAN_POINT('',(0.9,1.266106713614,0.));
#9413=CARTESIAN_POINT('',(0.9,1.34328341716202,0.));
#9414=CARTESIAN_POINT('',(0.292382661757373,1.22257596919059,0.));
#9415=CARTESIAN_POINT('Ctrl Pts',(0.9,1.266106713614,1.20346441145891E-16));
#9416=CARTESIAN_POINT('Ctrl Pts',(0.697432754539207,1.25280566772398,-2.10387859372414E-8));
#9417=CARTESIAN_POINT('Ctrl Pts',(0.494894520889663,1.23831317328004,3.6654767345328E-12));
#9418=CARTESIAN_POINT('Ctrl Pts',(0.292382661757371,1.22257596919059,2.98331735103528E-16));
#9419=CARTESIAN_POINT('Ctrl Pts',(0.292382661757373,1.22257596919059,2.94902990916057E-17));
#9420=CARTESIAN_POINT('Ctrl Pts',(0.284469747869226,1.22196105627757,-8.65621238729993E-13));
#9421=CARTESIAN_POINT('Ctrl Pts',(0.276673396002317,1.22038240716686,-1.19564355630166E-6));
#9422=CARTESIAN_POINT('Ctrl Pts',(0.269153172408756,1.21792571627104,-1.29137975931779E-6));
#9423=CARTESIAN_POINT('Ctrl Pts',(0.264330998492885,1.21635041859408,-1.35276844214688E-6));
#9424=CARTESIAN_POINT('Ctrl Pts',(0.259622238853914,1.21441292414196,-1.0165784587106E-6));
#9425=CARTESIAN_POINT('Ctrl Pts',(0.255072584042237,1.21212521597766,-4.21167369976509E-7));
#9426=CARTESIAN_POINT('Ctrl Pts',(0.247984787860257,1.20856125126747,5.06409032217246E-7));
#9427=CARTESIAN_POINT('Ctrl Pts',(0.241364979299678,1.20419126978451,2.25366520907849E-6));
#9428=CARTESIAN_POINT('Ctrl Pts',(0.235375785094684,1.19908071490398,1.28723124315333E-6));
#9429=CARTESIAN_POINT('Ctrl Pts',(0.235058634311792,1.19881009144014,1.23605486142058E-6));
#9430=CARTESIAN_POINT('Ctrl Pts',(0.234743258170683,1.19853738091759,1.17639378419006E-6));
#9431=CARTESIAN_POINT('Ctrl Pts',(0.234429683218046,1.19826258967301,1.10742116603597E-6));
#9432=CARTESIAN_POINT('Ctrl Pts',(0.23095881299434,1.19522100506769,3.4398325561458E-7));
#9433=CARTESIAN_POINT('Ctrl Pts',(0.227708211416394,1.19192479473749,-1.52348441667556E-6));
#9434=CARTESIAN_POINT('Ctrl Pts',(0.224692430858345,1.18840300965977,-3.42436181452249E-6));
#9435=CARTESIAN_POINT('Ctrl Pts',(0.219522873151367,1.18236607466387,-6.68278702580898E-6));
#9436=CARTESIAN_POINT('Ctrl Pts',(0.21509942609515,1.17573654654733,-9.78259773483875E-6));
#9437=CARTESIAN_POINT('Ctrl Pts',(0.211478909386775,1.16867548752938,-1.04320859863301E-5));
#9438=CARTESIAN_POINT('Ctrl Pts',(0.20968494559888,1.16517673715679,-1.075390701291E-5));
#9439=CARTESIAN_POINT('Ctrl Pts',(0.208088728862602,1.16157146972622,-1.05358292927083E-5));
#9440=CARTESIAN_POINT('Ctrl Pts',(0.206701335101202,1.15787708229469,-9.83193564179307E-6));
#9441=CARTESIAN_POINT('Ctrl Pts',(0.203919119965097,1.15046852899383,-8.42037994342582E-6));
#9442=CARTESIAN_POINT('Ctrl Pts',(0.202003457218558,1.1427818296106,-4.88542801801716E-6));
#9443=CARTESIAN_POINT('Ctrl Pts',(0.201024541128784,1.13496408391561,-2.30807221316776E-6));
#9444=CARTESIAN_POINT('Ctrl Pts',(0.200529226009753,1.13100843574523,-1.00397341389412E-6));
#9445=CARTESIAN_POINT('Ctrl Pts',(0.200274469344113,1.12701892049093,-1.14168925800036E-11));
#9446=CARTESIAN_POINT('Ctrl Pts',(0.200274469199584,1.12301388185427,-1.43114686768087E-17));
#9447=CARTESIAN_POINT('',(-1.73234772679968E-18,1.12356026268968,4.53319947845445E-20));
#9448=CARTESIAN_POINT('',(0.,-1.4,0.));
#9449=CARTESIAN_POINT('',(0.276326924564679,1.42224670711126,-2.77555756156289E-17));
#9450=CARTESIAN_POINT('Ctrl Pts',(0.276326924564681,1.42224670711126,-1.50920942409982E-16));
#9451=CARTESIAN_POINT('Ctrl Pts',(0.258529852003869,1.4208638358667,-3.32972379743633E-13));
#9452=CARTESIAN_POINT('Ctrl Pts',(0.240927013527826,1.41785398988725,-1.99727536601662E-6));
#9453=CARTESIAN_POINT('Ctrl Pts',(0.223720619657732,1.41333325652174,-2.71091968639774E-6));
#9454=CARTESIAN_POINT('Ctrl Pts',(0.206313289378911,1.40875972999491,-3.432897951005E-6));
#9455=CARTESIAN_POINT('Ctrl Pts',(0.18931019325249,1.40263932318529,-2.78724979559428E-6));
#9456=CARTESIAN_POINT('Ctrl Pts',(0.172932985028856,1.39504220432096,-6.31841720307455E-7));
#9457=CARTESIAN_POINT('Ctrl Pts',(0.170060146426803,1.39370954151055,-2.53746782677961E-7));
#9458=CARTESIAN_POINT('Ctrl Pts',(0.167206630967902,1.39233132643846,1.61597591574489E-7));
#9459=CARTESIAN_POINT('Ctrl Pts',(0.164373729059928,1.39090779908693,6.02790108062464E-7));
#9460=CARTESIAN_POINT('Ctrl Pts',(0.148213121449433,1.38278712717586,3.11962244863226E-6));
#9461=CARTESIAN_POINT('Ctrl Pts',(0.132864864406694,1.37326763401578,6.8005293729143E-6));
#9462=CARTESIAN_POINT('Ctrl Pts',(0.118540368157823,1.36244192017091,7.47011412280372E-6));
#9463=CARTESIAN_POINT('Ctrl Pts',(0.1130124780146,1.35826422653222,7.72851001154276E-6));
#9464=CARTESIAN_POINT('Ctrl Pts',(0.107637267132642,1.35389150739715,7.50091387420595E-6));
#9465=CARTESIAN_POINT('Ctrl Pts',(0.102427993107927,1.34932731552598,6.39696583889361E-6));
#9466=CARTESIAN_POINT('Ctrl Pts',(0.0920147884934566,1.34020361352282,4.19020214765608E-6));
#9467=CARTESIAN_POINT('Ctrl Pts',(0.082263696775192,1.33031540618347,-1.43705507633734E-6));
#9468=CARTESIAN_POINT('Ctrl Pts',(0.0732179607829324,1.31975004019149,-7.24116446069057E-6));
#9469=CARTESIAN_POINT('Ctrl Pts',(0.0614369648181435,1.30598990677343,-1.48003270644599E-5));
#9470=CARTESIAN_POINT('Ctrl Pts',(0.0509520748529884,1.29120077200215,-2.24515165560165E-5));
#9471=CARTESIAN_POINT('Ctrl Pts',(0.0418305631051555,1.27560026299671,-2.64881615939377E-5));
#9472=CARTESIAN_POINT('Ctrl Pts',(0.0329966685655992,1.26049166530727,-3.03975241584371E-5));
#9473=CARTESIAN_POINT('Ctrl Pts',(0.0254411283904758,1.24462062939249,-3.09701348507133E-5));
#9474=CARTESIAN_POINT('Ctrl Pts',(0.0192647836588538,1.2281607987719,-2.81763116144976E-5));
#9475=CARTESIAN_POINT('Ctrl Pts',(0.0129258683931997,1.2112677210496,-2.53089508159798E-5));
#9476=CARTESIAN_POINT('Ctrl Pts',(0.00809110271874438,1.19389182855556,
-1.89493195503086E-5));
#9477=CARTESIAN_POINT('Ctrl Pts',(0.00484442764459327,1.17622983835018,
-1.25518552566888E-5));
#9478=CARTESIAN_POINT('Ctrl Pts',(0.00165723550742335,1.1588914367474,-6.27160009448058E-6));
#9479=CARTESIAN_POINT('Ctrl Pts',(1.90718451428807E-9,1.14127598190669,
-1.51296892603399E-10));
#9480=CARTESIAN_POINT('Ctrl Pts',(2.41777084464267E-17,1.12356026268968,
-3.46944695195361E-18));
#9481=CARTESIAN_POINT('',(10.5166159648474,1.4155315881283,0.));
#9482=CARTESIAN_POINT('Ctrl Pts',(0.276326924564679,1.42224670711126,0.));
#9483=CARTESIAN_POINT('Ctrl Pts',(3.68975660465893,1.68747752195839,0.));
#9484=CARTESIAN_POINT('Ctrl Pts',(7.10318628475318,1.599994843061,0.));
#9485=CARTESIAN_POINT('Ctrl Pts',(10.5166159648474,1.4155315881283,0.));
#9486=CARTESIAN_POINT('',(10.8,1.11638029377732,-5.56631991785941E-17));
#9487=CARTESIAN_POINT('Ctrl Pts',(10.8,1.11638029377732,2.32452945780892E-16));
#9488=CARTESIAN_POINT('Ctrl Pts',(10.7999999994302,1.13421844616111,-9.29296349749781E-12));
#9489=CARTESIAN_POINT('Ctrl Pts',(10.7983603663884,1.15198349698667,-2.38856955364628E-6));
#9490=CARTESIAN_POINT('Ctrl Pts',(10.7951843826221,1.16946861094468,-3.77014304120448E-6));
#9491=CARTESIAN_POINT('Ctrl Pts',(10.7919669771209,1.18718176881198,-5.16973525142236E-6));
#9492=CARTESIAN_POINT('Ctrl Pts',(10.7871724978816,1.20460918321158,-5.4755482503851E-6));
#9493=CARTESIAN_POINT('Ctrl Pts',(10.7808573412527,1.22152732075962,-4.27334038376583E-6));
#9494=CARTESIAN_POINT('Ctrl Pts',(10.7797421066656,1.22451500471617,-4.06103467663179E-6));
#9495=CARTESIAN_POINT('Ctrl Pts',(10.7785793293545,1.22748675045939,-3.81081650224554E-6));
#9496=CARTESIAN_POINT('Ctrl Pts',(10.7773691713543,1.23044124224994,-3.53261416912234E-6));
#9497=CARTESIAN_POINT('Ctrl Pts',(10.7705159051166,1.24717287467681,-1.95712183132163E-6));
#9498=CARTESIAN_POINT('Ctrl Pts',(10.7622076549587,1.26320448426569,8.50150473021234E-7));
#9499=CARTESIAN_POINT('Ctrl Pts',(10.7525236566209,1.27832128496499,1.09915986206012E-6));
#9500=CARTESIAN_POINT('Ctrl Pts',(10.7482509716548,1.28499098118248,1.20902550183604E-6));
#9501=CARTESIAN_POINT('Ctrl Pts',(10.7437098328292,1.29148238441373,7.76315258636623E-7));
#9502=CARTESIAN_POINT('Ctrl Pts',(10.7389041877712,1.29777551763099,-7.54184826032082E-7));
#9503=CARTESIAN_POINT('Ctrl Pts',(10.7310976851069,1.30799836193882,-3.24039694621926E-6));
#9504=CARTESIAN_POINT('Ctrl Pts',(10.7225935645301,1.31769858917671,-8.57388820182801E-6));
#9505=CARTESIAN_POINT('Ctrl Pts',(10.7134588931078,1.3268364513864,-1.41086939541967E-5));
#9506=CARTESIAN_POINT('Ctrl Pts',(10.7004433550849,1.33985653580309,-2.19949628070403E-5));
#9507=CARTESIAN_POINT('Ctrl Pts',(10.6862650266646,1.35162127070648,-3.0022236679635E-5));
#9508=CARTESIAN_POINT('Ctrl Pts',(10.6711476119081,1.36204513612776,-3.40981369893719E-5));
#9509=CARTESIAN_POINT('Ctrl Pts',(10.6560301971515,1.37246900154903,-3.81740372991087E-5));
#9510=CARTESIAN_POINT('Ctrl Pts',(10.6399721826852,1.38155285075117,-3.83332859284948E-5));
#9511=CARTESIAN_POINT('Ctrl Pts',(10.6231652498763,1.38916602817047,-3.45204725343976E-5));
#9512=CARTESIAN_POINT('Ctrl Pts',(10.6063487480974,1.39678354012646,-3.07054883279539E-5));
#9513=CARTESIAN_POINT('Ctrl Pts',(10.5889271210941,1.40286310406803,-2.29928881382306E-5));
#9514=CARTESIAN_POINT('Ctrl Pts',(10.5711041279812,1.40730078588308,-1.53078138731408E-5));
#9515=CARTESIAN_POINT('Ctrl Pts',(10.5532811348684,1.41173846769814,-7.6227396080509E-6));
#9516=CARTESIAN_POINT('Ctrl Pts',(10.5350552605908,1.41453511891929,-9.16729947674095E-11));
#9517=CARTESIAN_POINT('Ctrl Pts',(10.5166159648474,1.4155315881283,2.48932818802672E-16));
#9518=CARTESIAN_POINT('',(10.8,-1.11638029377732,-1.39157997946485E-17));
#9519=CARTESIAN_POINT('',(10.8,1.4,0.));
#9520=CARTESIAN_POINT('',(10.5166159648474,-1.4155315881283,2.77555756156289E-17));
#9521=CARTESIAN_POINT('Ctrl Pts',(10.5166159648474,-1.4155315881283,-1.94289029309402E-16));
#9522=CARTESIAN_POINT('Ctrl Pts',(10.5344251606169,-1.41456917089032,1.72780596414851E-12));
#9523=CARTESIAN_POINT('Ctrl Pts',(10.5520727686739,-1.41197333457428,-2.53403886306205E-6));
#9524=CARTESIAN_POINT('Ctrl Pts',(10.5693578805681,-1.40785843881911,-4.04156906196095E-6));
#9525=CARTESIAN_POINT('Ctrl Pts',(10.5868701251756,-1.40368947182374,-5.56890876087065E-6));
#9526=CARTESIAN_POINT('Ctrl Pts',(10.604011804524,-1.39796079212135,-5.98742339745246E-6));
#9527=CARTESIAN_POINT('Ctrl Pts',(10.6205627760847,-1.39074087128671,-4.81856832951796E-6));
#9528=CARTESIAN_POINT('Ctrl Pts',(10.6234754753687,-1.38947028374636,-4.61286902618664E-6));
#9529=CARTESIAN_POINT('Ctrl Pts',(10.6263698187278,-1.38815339768352,-4.36721670635639E-6));
#9530=CARTESIAN_POINT('Ctrl Pts',(10.629244514885,-1.38679044403738,-4.09122931699412E-6));
#9531=CARTESIAN_POINT('Ctrl Pts',(10.6455827855986,-1.37904412775797,-2.5226612199239E-6));
#9532=CARTESIAN_POINT('Ctrl Pts',(10.6611432679573,-1.36988219838444,3.58605122725343E-7));
#9533=CARTESIAN_POINT('Ctrl Pts',(10.6757157985124,-1.35939560704671,7.40589063327193E-7));
#9534=CARTESIAN_POINT('Ctrl Pts',(10.6821516119741,-1.35476430808026,9.09288478831296E-7));
#9535=CARTESIAN_POINT('Ctrl Pts',(10.6883944859408,-1.34987400891586,5.44816430868337E-7));
#9536=CARTESIAN_POINT('Ctrl Pts',(10.6944246343503,-1.34472976213865,-9.14752338109426E-7));
#9537=CARTESIAN_POINT('Ctrl Pts',(10.7041966733629,-1.33639335368171,-3.28002794718031E-6));
#9538=CARTESIAN_POINT('Ctrl Pts',(10.7134106653983,-1.3273903805878,-8.47259327327479E-6));
#9539=CARTESIAN_POINT('Ctrl Pts',(10.7220307555455,-1.31778973409553,-1.38734771921913E-5));
#9540=CARTESIAN_POINT('Ctrl Pts',(10.7343338492722,-1.3040871333553,-2.15819326638919E-5));
#9541=CARTESIAN_POINT('Ctrl Pts',(10.7453199276401,-1.28929041974124,-2.94555326738194E-5));
#9542=CARTESIAN_POINT('Ctrl Pts',(10.7549158277293,-1.27362793268665,-3.3443536645081E-5));
#9543=CARTESIAN_POINT('Ctrl Pts',(10.7645117278185,-1.25796544563206,-3.74315406163426E-5));
#9544=CARTESIAN_POINT('Ctrl Pts',(10.7727182208071,-1.24143562566754,-3.75750290962259E-5));
#9545=CARTESIAN_POINT('Ctrl Pts',(10.7794153247677,-1.22423716044977,-3.38265125308188E-5));
#9546=CARTESIAN_POINT('Ctrl Pts',(10.7861166764432,-1.20702778690835,-3.00756184258222E-5));
#9547=CARTESIAN_POINT('Ctrl Pts',(10.7912490477072,-1.18929683429644,-2.25107044755726E-5));
#9548=CARTESIAN_POINT('Ctrl Pts',(10.7947196858669,-1.17125359626911,-1.49815203503087E-5));
#9549=CARTESIAN_POINT('Ctrl Pts',(10.7981903240266,-1.15321035824179,-7.45233622504479E-6));
#9550=CARTESIAN_POINT('Ctrl Pts',(10.7999999985278,-1.13485327409571,-1.17780195603766E-10));
#9551=CARTESIAN_POINT('Ctrl Pts',(10.8,-1.11638029377732,-1.38777878078145E-17));
#9552=CARTESIAN_POINT('',(0.276326924564679,-1.42224670711126,-5.55111512312578E-17));
#9553=CARTESIAN_POINT('Ctrl Pts',(10.5166159648474,-1.4155315881283,0.));
#9554=CARTESIAN_POINT('Ctrl Pts',(7.10318628475318,-1.599994843061,0.));
#9555=CARTESIAN_POINT('Ctrl Pts',(3.68975660465893,-1.68747752195839,0.));
#9556=CARTESIAN_POINT('Ctrl Pts',(0.276326924564679,-1.42224670711126,0.));
#9557=CARTESIAN_POINT('',(-7.25311916552711E-19,-1.12356026268968,1.39157997946485E-17));
#9558=CARTESIAN_POINT('Ctrl Pts',(1.80411241501588E-16,-1.12356026268968,
-1.53523027623947E-16));
#9559=CARTESIAN_POINT('Ctrl Pts',(7.41078168374529E-10,-1.14141522098415,
-1.3067981184062E-11));
#9560=CARTESIAN_POINT('Ctrl Pts',(0.00163694718329378,-1.15920272117896,
-1.78823819589733E-6));
#9561=CARTESIAN_POINT('Ctrl Pts',(0.00481087395297265,-1.17671209893291,
-2.3181425555783E-6));
#9562=CARTESIAN_POINT('Ctrl Pts',(0.00802138847203439,-1.19442331774104,
-2.85415543927884E-6));
#9563=CARTESIAN_POINT('Ctrl Pts',(0.0128049030182357,-1.21185152247087,
-2.04128886843626E-6));
#9564=CARTESIAN_POINT('Ctrl Pts',(0.0191087770915565,-1.22877027194193,
1.71240493184593E-7));
#9565=CARTESIAN_POINT('Ctrl Pts',(0.0202201941454154,-1.23175316571065,
5.613248819379E-7));
#9566=CARTESIAN_POINT('Ctrl Pts',(0.0213789882593307,-1.23472016785247,
9.85829603970989E-7));
#9567=CARTESIAN_POINT('Ctrl Pts',(0.0225850188675993,-1.23766995297306,
1.43287414332239E-6));
#9568=CARTESIAN_POINT('Ctrl Pts',(0.0294291562303479,-1.25440977235863,
3.96981990042924E-6));
#9569=CARTESIAN_POINT('Ctrl Pts',(0.0377300686697735,-1.27044838970616,
7.55798501181421E-6));
#9570=CARTESIAN_POINT('Ctrl Pts',(0.0474121614036163,-1.28556782977674,
8.05058320302158E-6));
#9571=CARTESIAN_POINT('Ctrl Pts',(0.0511425121829324,-1.29139310088294,
8.24037316857697E-6));
#9572=CARTESIAN_POINT('Ctrl Pts',(0.0550784035723718,-1.29708174651376,
7.93435480917585E-6));
#9573=CARTESIAN_POINT('Ctrl Pts',(0.0592173503759339,-1.30262033374061,
6.74858081742264E-6));
#9574=CARTESIAN_POINT('Ctrl Pts',(0.0675201807396794,-1.31373087764993,
4.36988865960166E-6));
#9575=CARTESIAN_POINT('Ctrl Pts',(0.0766394565597649,-1.32423847988766,
-1.46587651676554E-6));
#9576=CARTESIAN_POINT('Ctrl Pts',(0.0864911062490747,-1.33409287340636,
-7.46705500292641E-6));
#9577=CARTESIAN_POINT('Ctrl Pts',(0.0992988409846585,-1.34690417528452,
-1.52689465211603E-5));
#9578=CARTESIAN_POINT('Ctrl Pts',(0.113232871116931,-1.35850278376499,-2.31308069859054E-5));
#9579=CARTESIAN_POINT('Ctrl Pts',(0.128081622025101,-1.36880445085772,-2.72849174168177E-5));
#9580=CARTESIAN_POINT('Ctrl Pts',(0.142447925282442,-1.37877140864598,-3.13040575171566E-5));
#9581=CARTESIAN_POINT('Ctrl Pts',(0.157671864768995,-1.38752483454192,-3.1899138628041E-5));
#9582=CARTESIAN_POINT('Ctrl Pts',(0.173588691395025,-1.39495074934422,-2.90326641197332E-5));
#9583=CARTESIAN_POINT('Ctrl Pts',(0.189936400238013,-1.40257769006131,-2.60885916756054E-5));
#9584=CARTESIAN_POINT('Ctrl Pts',(0.206881864105471,-1.40874232120582,-1.95409011442111E-5));
#9585=CARTESIAN_POINT('Ctrl Pts',(0.22423558959196,-1.41334558507228,-1.29462590315495E-5));
#9586=CARTESIAN_POINT('Ctrl Pts',(0.241260467995769,-1.4178616186841,-6.47658310103417E-6));
#9587=CARTESIAN_POINT('Ctrl Pts',(0.258679581942429,-1.42087546890512,-1.12101563992788E-10));
#9588=CARTESIAN_POINT('Ctrl Pts',(0.27632692456468,-1.42224670711126,1.05818132034585E-16));
#9589=CARTESIAN_POINT('',(0.,-1.4,0.));
#9590=CARTESIAN_POINT('',(0.292382661757373,-1.22257596919059,0.));
#9591=CARTESIAN_POINT('Ctrl Pts',(0.200274469199584,-1.12301388185427,-2.68882138776405E-17));
#9592=CARTESIAN_POINT('Ctrl Pts',(0.200274469314753,-1.13095194822878,-2.85686379674833E-12));
#9593=CARTESIAN_POINT('Ctrl Pts',(0.201244085522878,-1.13884856843413,-1.08105759021766E-6));
#9594=CARTESIAN_POINT('Ctrl Pts',(0.203110344361254,-1.14653799330522,-1.10782444979703E-6));
#9595=CARTESIAN_POINT('Ctrl Pts',(0.204308287281872,-1.15147379958167,-1.12500597321754E-6));
#9596=CARTESIAN_POINT('Ctrl Pts',(0.205876831658669,-1.15632444796435,-7.573778542164E-7));
#9597=CARTESIAN_POINT('Ctrl Pts',(0.207807574899602,-1.16104329283393,-1.57887042599725E-7));
#9598=CARTESIAN_POINT('Ctrl Pts',(0.21096922807971,-1.1687705506961,8.23798139982571E-7));
#9599=CARTESIAN_POINT('Ctrl Pts',(0.215060220496011,-1.17605061753432,2.67511715935828E-6));
#9600=CARTESIAN_POINT('Ctrl Pts',(0.220020901709485,-1.18268777995331,1.20301732358232E-6));
#9601=CARTESIAN_POINT('Ctrl Pts',(0.222788929945646,-1.18639127392786,3.81595076007225E-7));
#9602=CARTESIAN_POINT('Ctrl Pts',(0.225828882930032,-1.18989419630164,-1.55522758636672E-6));
#9603=CARTESIAN_POINT('Ctrl Pts',(0.229112809647272,-1.19317965616817,-3.52099818518546E-6));
#9604=CARTESIAN_POINT('Ctrl Pts',(0.234731790749985,-1.1988012605745,-6.88454091865859E-6));
#9605=CARTESIAN_POINT('Ctrl Pts',(0.240999377733319,-1.20372479786492,-1.00686973618824E-5));
#9606=CARTESIAN_POINT('Ctrl Pts',(0.247759525934523,-1.2078808899968,-1.07387199666626E-5));
#9607=CARTESIAN_POINT('Ctrl Pts',(0.251104201987095,-1.20993717358883,-1.10702228411842E-5));
#9608=CARTESIAN_POINT('Ctrl Pts',(0.254570062984725,-1.21180502729412,-1.08478245319173E-5));
#9609=CARTESIAN_POINT('Ctrl Pts',(0.258140701417296,-1.21347208138814,-1.01264154182862E-5));
#9610=CARTESIAN_POINT('Ctrl Pts',(0.265309933881728,-1.21681924144269,-8.67794906268977E-6));
#9611=CARTESIAN_POINT('Ctrl Pts',(0.27282354441991,-1.21932394229889,-5.03816435877804E-6));
#9612=CARTESIAN_POINT('Ctrl Pts',(0.280540402387729,-1.22090470300999,-2.38011023443526E-6));
#9613=CARTESIAN_POINT('Ctrl Pts',(0.284441227387562,-1.22170376798259,-1.03647996128718E-6));
#9614=CARTESIAN_POINT('Ctrl Pts',(0.288394358015454,-1.22226603782358,-8.41267709508591E-12));
#9615=CARTESIAN_POINT('Ctrl Pts',(0.292382661757373,-1.22257596919059,3.10081821330854E-17));
#9616=CARTESIAN_POINT('',(0.9,-1.266106713614,0.));
#9617=CARTESIAN_POINT('Ctrl Pts',(0.29238266175737,-1.22257596919059,3.4274341177698E-16));
#9618=CARTESIAN_POINT('Ctrl Pts',(0.494894519961671,-1.23831317320793,3.6654050078524E-12));
#9619=CARTESIAN_POINT('Ctrl Pts',(0.697432753591781,-1.25280566766171,-2.10377631034678E-8));
#9620=CARTESIAN_POINT('Ctrl Pts',(0.900000000000002,-1.266106713614,4.80511808774455E-17));
#9621=CARTESIAN_POINT('',(0.9,1.34328341716202,0.));
#9622=CARTESIAN_POINT('',(3.5,-1.37552980833516,0.));
#9623=CARTESIAN_POINT('Ctrl Pts',(1.10000000028363,-1.27885335028943,-5.13283219638443E-11));
#9624=CARTESIAN_POINT('Ctrl Pts',(1.8994825293422,-1.32827224294784,2.51289069808066E-7));
#9625=CARTESIAN_POINT('Ctrl Pts',(2.69943073922525,-1.35940904940056,2.35357980118634E-7));
#9626=CARTESIAN_POINT('Ctrl Pts',(3.50000000097418,-1.37552980835478,8.59034485311056E-16));
#9627=CARTESIAN_POINT('',(3.5,1.44777777777778,0.));
#9628=CARTESIAN_POINT('',(7.1,-1.35793097395724,0.));
#9629=CARTESIAN_POINT('Ctrl Pts',(3.700000000362,-1.379246395385,-6.25385501848083E-12));
#9630=CARTESIAN_POINT('Ctrl Pts',(4.26467016042339,-1.38886773733237,1.63880713394601E-8));
#9631=CARTESIAN_POINT('Ctrl Pts',(4.82965558050887,-1.39115503781354,-4.12727732537403E-8));
#9632=CARTESIAN_POINT('Ctrl Pts',(5.39500817395676,-1.38725486475042,-3.97626883737645E-8));
#9633=CARTESIAN_POINT('Ctrl Pts',(5.96336684492344,-1.38333395379258,-3.82445741104923E-8));
#9634=CARTESIAN_POINT('Ctrl Pts',(6.53173538886785,-1.37316170188981,3.71969681223073E-9));
#9635=CARTESIAN_POINT('Ctrl Pts',(7.1000000000396,-1.35793097389613,-4.88946831112289E-12));
#9636=CARTESIAN_POINT('',(7.1,1.42555555555556,0.));
#9637=CARTESIAN_POINT('',(10.2,-1.23178301601145,0.));
#9638=CARTESIAN_POINT('',(10.5052647440597,-1.21555035534119,0.));
#9639=CARTESIAN_POINT('Ctrl Pts',(10.2,-1.23178301601145,-4.56855690431079E-17));
#9640=CARTESIAN_POINT('Ctrl Pts',(10.3017652114452,-1.22646242153193,-6.28718440835499E-11));
#9641=CARTESIAN_POINT('Ctrl Pts',(10.4035203469111,-1.22104923788321,1.43982679105611E-13));
#9642=CARTESIAN_POINT('Ctrl Pts',(10.5052647440597,-1.21555035534119,6.44897004721534E-17));
#9643=CARTESIAN_POINT('',(10.5997255308004,-1.11583328740478,1.38777878078145E-17));
#9644=CARTESIAN_POINT('Ctrl Pts',(10.5052647440597,-1.21555035534119,-1.86482773667507E-17));
#9645=CARTESIAN_POINT('Ctrl Pts',(10.5131888530666,-1.21512208850275,-5.60416335832109E-13));
#9646=CARTESIAN_POINT('Ctrl Pts',(10.5210180054001,-1.21372544600509,-1.35972994235015E-6));
#9647=CARTESIAN_POINT('Ctrl Pts',(10.5285917824072,-1.2114444991589,-1.66070161277884E-6));
#9648=CARTESIAN_POINT('Ctrl Pts',(10.5334522234388,-1.20998071066451,-1.8538489757029E-6));
#9649=CARTESIAN_POINT('Ctrl Pts',(10.538207639053,-1.20815156029678,-1.66445033219183E-6));
#9650=CARTESIAN_POINT('Ctrl Pts',(10.542812250732,-1.20596855068549,-1.19054254011085E-6));
#9651=CARTESIAN_POINT('Ctrl Pts',(10.5499808226381,-1.20256998801374,-4.52751316616249E-7));
#9652=CARTESIAN_POINT('Ctrl Pts',(10.5567010840309,-1.19835579238971,1.16775294480959E-6));
#9653=CARTESIAN_POINT('Ctrl Pts',(10.5628099082467,-1.1933896765605,3.12218506849373E-7));
#9654=CARTESIAN_POINT('Ctrl Pts',(10.563392699667,-1.1929159013142,2.30599178383296E-7));
#9655=CARTESIAN_POINT('Ctrl Pts',(10.563969906567,-1.19243524850296,1.23643260424227E-7));
#9656=CARTESIAN_POINT('Ctrl Pts',(10.5645413730323,-1.19194775268147,-1.33988689923433E-8));
#9657=CARTESIAN_POINT('Ctrl Pts',(10.5677990734116,-1.18916873515523,-7.94620907596477E-7));
#9658=CARTESIAN_POINT('Ctrl Pts',(10.5708705204042,-1.18616755700159,-2.52696578471864E-6));
#9659=CARTESIAN_POINT('Ctrl Pts',(10.5737438185805,-1.18296717200411,-4.3349897000341E-6));
#9660=CARTESIAN_POINT('Ctrl Pts',(10.579054042416,-1.17705244973962,-7.67644996655303E-6));
#9661=CARTESIAN_POINT('Ctrl Pts',(10.5836289246435,-1.17052745137283,-1.0999028846932E-5));
#9662=CARTESIAN_POINT('Ctrl Pts',(10.5874112735695,-1.16355342251842,-1.18035167459916E-5));
#9663=CARTESIAN_POINT('Ctrl Pts',(10.5894705469099,-1.15975646143,-1.22415145393192E-5));
#9664=CARTESIAN_POINT('Ctrl Pts',(10.5912942421259,-1.15582570378367,-1.20038889321768E-5));
#9665=CARTESIAN_POINT('Ctrl Pts',(10.5928674986933,-1.15178403025788,-1.11465830745351E-5));
#9666=CARTESIAN_POINT('Ctrl Pts',(10.5957384082276,-1.14440870489779,-9.58215448007377E-6));
#9667=CARTESIAN_POINT('Ctrl Pts',(10.5977463817932,-1.13674651935037,-5.80208140981121E-6));
#9668=CARTESIAN_POINT('Ctrl Pts',(10.5988207707371,-1.12894377506163,-2.8960211281105E-6));
#9669=CARTESIAN_POINT('Ctrl Pts',(10.5994175893465,-1.12460938291963,-1.28171667533415E-6));
#9670=CARTESIAN_POINT('Ctrl Pts',(10.5997255306822,-1.12023121224821,-9.4020583932734E-12));
#9671=CARTESIAN_POINT('Ctrl Pts',(10.5997255308004,-1.11583328740478,-9.97465998686664E-18));
#9672=CARTESIAN_POINT('',(10.5997255308004,1.11583328740478,0.));
#9673=CARTESIAN_POINT('',(10.5997255308004,0.7,0.));
#9674=CARTESIAN_POINT('',(10.5052647440597,1.21555035534119,0.));
#9675=CARTESIAN_POINT('Ctrl Pts',(10.5997255308004,1.11583328740478,8.8037216405823E-17));
#9676=CARTESIAN_POINT('Ctrl Pts',(10.5997255307124,1.12376989384288,-2.22024716398596E-12));
#9677=CARTESIAN_POINT('Ctrl Pts',(10.5987536115518,1.13166401228391,-1.27532141444775E-6));
#9678=CARTESIAN_POINT('Ctrl Pts',(10.5968849989732,1.13935090273995,-1.5236651967046E-6));
#9679=CARTESIAN_POINT('Ctrl Pts',(10.5956849616024,1.14428748291596,-1.68315348385219E-6));
#9680=CARTESIAN_POINT('Ctrl Pts',(10.5941139374364,1.14913880701507,-1.46899737395989E-6));
#9681=CARTESIAN_POINT('Ctrl Pts',(10.5921809408638,1.1538584293407,-9.90118991603547E-7));
#9682=CARTESIAN_POINT('Ctrl Pts',(10.5891742477341,1.16119959911942,-2.45244239835432E-7));
#9683=CARTESIAN_POINT('Ctrl Pts',(10.5853292249979,1.16813727090899,1.33309554558619E-6));
#9684=CARTESIAN_POINT('Ctrl Pts',(10.5807005079991,1.17450509276749,4.08358240744415E-7));
#9685=CARTESIAN_POINT('Ctrl Pts',(10.5802604812716,1.17511044665166,3.20448539159982E-7));
#9686=CARTESIAN_POINT('Ctrl Pts',(10.5798133373602,1.17571063303672,2.07176952714776E-7));
#9687=CARTESIAN_POINT('Ctrl Pts',(10.5793591019426,1.17630549598644,6.38823567561716E-8));
#9688=CARTESIAN_POINT('Ctrl Pts',(10.5767566952267,1.17971358631841,-7.57081408668461E-7));
#9689=CARTESIAN_POINT('Ctrl Pts',(10.5739217504488,1.18294722379721,-2.53660858190298E-6));
#9690=CARTESIAN_POINT('Ctrl Pts',(10.570876618072,1.18599321478588,-4.38998728286835E-6));
#9691=CARTESIAN_POINT('Ctrl Pts',(10.5652565693637,1.19161484813492,-7.81055403847458E-6));
#9692=CARTESIAN_POINT('Ctrl Pts',(10.5589874561388,1.19653507038546,-1.11999964534866E-5));
#9693=CARTESIAN_POINT('Ctrl Pts',(10.5522271124844,1.20068789486255,-1.20263298844839E-5));
#9694=CARTESIAN_POINT('Ctrl Pts',(10.5485500617744,1.20294667739977,-1.24757848359648E-5));
#9695=CARTESIAN_POINT('Ctrl Pts',(10.5447269560479,1.20497781184918,-1.22374322375965E-5));
#9696=CARTESIAN_POINT('Ctrl Pts',(10.5407797717187,1.20676523914267,-1.13674773191707E-5));
#9697=CARTESIAN_POINT('Ctrl Pts',(10.5335711832013,1.210029547771,-9.77871264224002E-6));
#9698=CARTESIAN_POINT('Ctrl Pts',(10.5260296312848,1.21244761587922,-5.9245235663186E-6));
#9699=CARTESIAN_POINT('Ctrl Pts',(10.5182973307397,1.21394093281975,-2.95733858081469E-6));
#9700=CARTESIAN_POINT('Ctrl Pts',(10.514004731837,1.21476995008607,-1.31010113336685E-6));
#9701=CARTESIAN_POINT('Ctrl Pts',(10.5096528988527,1.21531319279956,-7.28166367327128E-12));
#9702=CARTESIAN_POINT('Ctrl Pts',(10.5052647440597,1.21555035534119,-3.31765864780564E-17));
#9703=CARTESIAN_POINT('',(10.2,1.23178301601145,0.));
#9704=CARTESIAN_POINT('Ctrl Pts',(10.5052647440597,1.21555035534119,1.20285454773689E-16));
#9705=CARTESIAN_POINT('Ctrl Pts',(10.4035203468995,1.22104923788384,1.44021921739714E-13));
#9706=CARTESIAN_POINT('Ctrl Pts',(10.3017652114309,1.22646242153268,-6.28696045710378E-11));
#9707=CARTESIAN_POINT('Ctrl Pts',(10.2,1.23178301601145,1.23125603768043E-16));
#9708=CARTESIAN_POINT('',(10.2,-1.30754691548544,0.));
#9709=CARTESIAN_POINT('Origin',(8.8,0.,0.));
#9710=CARTESIAN_POINT('',(8.4,-4.89858719658942E-17,0.));
#9711=CARTESIAN_POINT('Origin',(2.,0.,0.));
#9712=CARTESIAN_POINT('',(1.6,-4.89858719658941E-17,0.7));
#9713=CARTESIAN_POINT('Origin',(2.,0.,0.7));
#9714=CARTESIAN_POINT('',(1.6,-4.89858719658941E-17,0.));
#9715=CARTESIAN_POINT('Origin',(10.2,-1.30754691548544,0.));
#9716=CARTESIAN_POINT('',(10.1999999975107,-1.19856231453552,0.605472757505173));
#9717=CARTESIAN_POINT('Ctrl Pts',(10.2,-1.23178301601145,0.));
#9718=CARTESIAN_POINT('Ctrl Pts',(10.2,-1.22625045235593,0.100869147801815));
#9719=CARTESIAN_POINT('Ctrl Pts',(10.2,-1.22071692450357,0.201739022585575));
#9720=CARTESIAN_POINT('Ctrl Pts',(10.2,-1.2096433936729,0.403562754186249));
#9721=CARTESIAN_POINT('Ctrl Pts',(10.1999999975107,-1.20410330368611,0.50451817268257));
#9722=CARTESIAN_POINT('Ctrl Pts',(10.1999999975107,-1.19856231453552,0.605472757505173));
#9723=CARTESIAN_POINT('',(10.1999999975107,1.19856231453552,0.605472757505173));
#9724=CARTESIAN_POINT('Ctrl Pts',(10.1999999975107,1.19856231453552,0.605472757505173));
#9725=CARTESIAN_POINT('Ctrl Pts',(10.1999999975107,1.20410418062036,0.504502195294633));
#9726=CARTESIAN_POINT('Ctrl Pts',(10.2,1.20964514726505,0.403530798997214));
#9727=CARTESIAN_POINT('Ctrl Pts',(10.2,1.22071867750565,0.201707067365009));
#9728=CARTESIAN_POINT('Ctrl Pts',(10.2,1.22625132869937,0.100853170395858));
#9729=CARTESIAN_POINT('Ctrl Pts',(10.2,1.23178301601145,0.));
#9730=CARTESIAN_POINT('',(10.1999999980542,1.09857320530976,0.7));
#9731=CARTESIAN_POINT('Ctrl Pts',(10.1999999999973,1.09857320510493,0.7));
#9732=CARTESIAN_POINT('Ctrl Pts',(10.2000000008642,1.10649088744708,0.699999999248278));
#9733=CARTESIAN_POINT('Ctrl Pts',(10.1999989363772,1.11434529358656,0.699006164779054));
#9734=CARTESIAN_POINT('Ctrl Pts',(10.1999980093114,1.12199598895487,0.697118997523365));
#9735=CARTESIAN_POINT('Ctrl Pts',(10.1999974900707,1.12628106973794,0.696062013320951));
#9736=CARTESIAN_POINT('Ctrl Pts',(10.1999970168623,1.13050229860485,0.694723760583242));
#9737=CARTESIAN_POINT('Ctrl Pts',(10.199996713894,1.13463332887353,0.693115046692397));
#9738=CARTESIAN_POINT('Ctrl Pts',(10.1999961690675,1.14206214329588,0.690222103243312));
#9739=CARTESIAN_POINT('Ctrl Pts',(10.1999962772589,1.14911941279843,0.686488866209959));
#9740=CARTESIAN_POINT('Ctrl Pts',(10.1999969599022,1.15565885618684,0.681996408643444));
#9741=CARTESIAN_POINT('Ctrl Pts',(10.1999973343062,1.15924549304116,0.679532465931891));
#9742=CARTESIAN_POINT('Ctrl Pts',(10.1999978674396,1.16267609380848,0.676839263748528));
#9743=CARTESIAN_POINT('Ctrl Pts',(10.1999983417863,1.16592263776853,0.673924718551186));
#9744=CARTESIAN_POINT('Ctrl Pts',(10.199998806773,1.16910511991263,0.671067684066867));
#9745=CARTESIAN_POINT('Ctrl Pts',(10.1999992207276,1.17209141256199,0.668015240668471));
#9746=CARTESIAN_POINT('Ctrl Pts',(10.1999992206607,1.17485880184773,0.664778864469812));
#9747=CARTESIAN_POINT('Ctrl Pts',(10.1999992205369,1.17997899231675,0.658790960038769));
#9748=CARTESIAN_POINT('Ctrl Pts',(10.1999979581638,1.18435276586188,0.652174799271591));
#9749=CARTESIAN_POINT('Ctrl Pts',(10.1999975326045,1.18791964688485,0.645095405674036));
#9750=CARTESIAN_POINT('Ctrl Pts',(10.1999974898604,1.18827791229431,0.644384335742179));
#9751=CARTESIAN_POINT('Ctrl Pts',(10.1999974535047,1.18862799840101,0.643668573506599));
#9752=CARTESIAN_POINT('Ctrl Pts',(10.1999974242393,1.18896981696374,0.64294827577739));
#9753=CARTESIAN_POINT('Ctrl Pts',(10.1999971329942,1.1923715530028,0.635779961907205));
#9754=CARTESIAN_POINT('Ctrl Pts',(10.1999977790614,1.19491900203126,0.628247233077589));
#9755=CARTESIAN_POINT('Ctrl Pts',(10.1999987199397,1.19655829940385,0.620518158911201));
#9756=CARTESIAN_POINT('Ctrl Pts',(10.1999993222661,1.19760773597399,0.615570201805241));
#9757=CARTESIAN_POINT('Ctrl Pts',(10.2,1.19828413277105,0.610541112135461));
#9758=CARTESIAN_POINT('Ctrl Pts',(10.2,1.19856231427281,0.60547275750556));
#9759=CARTESIAN_POINT('',(10.2,-1.09857320510402,0.7));
#9760=CARTESIAN_POINT('',(10.2,-0.653773457742722,0.7));
#9761=CARTESIAN_POINT('Ctrl Pts',(10.2,-1.19856231427281,0.60547275750556));
#9762=CARTESIAN_POINT('Ctrl Pts',(10.2,-1.19812809376428,0.613384079828744));
#9763=CARTESIAN_POINT('Ctrl Pts',(10.1999984889428,-1.1967261327477,0.621202329970501));
#9764=CARTESIAN_POINT('Ctrl Pts',(10.1999978161146,-1.19444079525024,0.628767398200536));
#9765=CARTESIAN_POINT('Ctrl Pts',(10.1999974438306,-1.19317629038787,0.632953241898348));
#9766=CARTESIAN_POINT('Ctrl Pts',(10.1999972759003,-1.19164034846853,0.637061602680377));
#9767=CARTESIAN_POINT('Ctrl Pts',(10.1999973648938,-1.18984073583679,0.641063423920242));
#9768=CARTESIAN_POINT('Ctrl Pts',(10.1999975257516,-1.18658789218766,0.648296813248274));
#9769=CARTESIAN_POINT('Ctrl Pts',(10.1999986492083,-1.18251199594868,0.655103972585077));
#9770=CARTESIAN_POINT('Ctrl Pts',(10.1999990866637,-1.1776776067306,0.66132208754656));
#9771=CARTESIAN_POINT('Ctrl Pts',(10.1999991692372,-1.17676507450965,0.662495809810115));
#9772=CARTESIAN_POINT('Ctrl Pts',(10.1999992204458,-1.17582538639523,0.663648473741297));
#9773=CARTESIAN_POINT('Ctrl Pts',(10.1999992199672,-1.17485880188435,0.664778864469789));
#9774=CARTESIAN_POINT('Ctrl Pts',(10.1999992190419,-1.17299032792757,0.666963987046661));
#9775=CARTESIAN_POINT('Ctrl Pts',(10.1999990265713,-1.17102137903347,0.669065925022507));
#9776=CARTESIAN_POINT('Ctrl Pts',(10.1999987631451,-1.16895889720817,0.671081139337088));
#9777=CARTESIAN_POINT('Ctrl Pts',(10.1999980371048,-1.16327440276409,0.676635357771578));
#9778=CARTESIAN_POINT('Ctrl Pts',(10.1999968952367,-1.15694629605269,0.681471105251756));
#9779=CARTESIAN_POINT('Ctrl Pts',(10.1999965193249,-1.15013861030111,0.685534582868085));
#9780=CARTESIAN_POINT('Ctrl Pts',(10.1999962798276,-1.14580136285465,0.688123466749966));
#9781=CARTESIAN_POINT('Ctrl Pts',(10.1999963003895,-1.14126848503633,0.690398200126003));
#9782=CARTESIAN_POINT('Ctrl Pts',(10.1999965837416,-1.13657664085124,0.692335536714198));
#9783=CARTESIAN_POINT('Ctrl Pts',(10.199997026059,-1.12925259320479,0.695359751696499));
#9784=CARTESIAN_POINT('Ctrl Pts',(10.1999981114625,-1.12162598460505,0.697529439192009));
#9785=CARTESIAN_POINT('Ctrl Pts',(10.1999989867727,-1.11384404680861,0.698775198878229));
#9786=CARTESIAN_POINT('Ctrl Pts',(10.1999995533653,-1.10880676031141,0.699581585232154));
#9787=CARTESIAN_POINT('Ctrl Pts',(10.200000000559,-1.10370379302489,0.699999999512891));
#9788=CARTESIAN_POINT('Ctrl Pts',(10.1999999999973,-1.09857320510493,0.7));
#9789=CARTESIAN_POINT('Ctrl Pts',(10.0273290644374,-1.24073895154929,-0.000342977371441382));
#9790=CARTESIAN_POINT('Ctrl Pts',(10.0182194939277,-1.2301570933055,0.201590462913323));
#9791=CARTESIAN_POINT('Ctrl Pts',(10.0091098064739,-1.21957524432673,0.403523898419685));
#9792=CARTESIAN_POINT('Ctrl Pts',(10.,-1.20899340483173,0.605457329065658));
#9793=CARTESIAN_POINT('Ctrl Pts',(9.11786336174441,-1.287320026752,-0.000205293215301774));
#9794=CARTESIAN_POINT('Ctrl Pts',(9.11054075262461,-1.27673792859995,0.201728409731728));
#9795=CARTESIAN_POINT('Ctrl Pts',(9.10321803982027,-1.2661558351744,0.403662109352091));
#9796=CARTESIAN_POINT('Ctrl Pts',(9.09589522044064,-1.25557375159922,0.605595805683776));
#9797=CARTESIAN_POINT('Ctrl Pts',(8.20875307681921,-1.32613868191631,-8.19769783003664E-5));
#9798=CARTESIAN_POINT('Ctrl Pts',(8.20321812688803,-1.31555630757271,0.201851960079368));
#9799=CARTESIAN_POINT('Ctrl Pts',(8.19768309032111,-1.30497393555236,0.403785895133155));
#9800=CARTESIAN_POINT('Ctrl Pts',(8.19214796413157,-1.29439157095064,0.605719828258773));
#9801=CARTESIAN_POINT('Ctrl Pts',(7.29999999999999,-1.35236351479115,1.04083408558608E-17));
#9802=CARTESIAN_POINT('Ctrl Pts',(7.29625341766944,-1.34178092325774,0.201934092022114));
#9803=CARTESIAN_POINT('Ctrl Pts',(7.2925067690755,-1.33119833465137,0.403868182971915));
#9804=CARTESIAN_POINT('Ctrl Pts',(7.28876005303739,-1.32061574904145,0.605802272831199));
#9805=CARTESIAN_POINT('Ctrl Pts',(7.29999999953094,-1.32031613471704,0.605285370449856));
#9806=CARTESIAN_POINT('Ctrl Pts',(8.20058408060299,-1.29406305600824,0.605326635812744));
#9807=CARTESIAN_POINT('Ctrl Pts',(9.10058974048747,-1.25534320916473,0.605388449123016));
#9808=CARTESIAN_POINT('Ctrl Pts',(9.99999999968202,-1.20899340489109,0.605457329065633));
#9809=CARTESIAN_POINT('Ctrl Pts',(10.5052670937641,-1.21555282972197,-4.72190879230918E-5));
#9810=CARTESIAN_POINT('Ctrl Pts',(10.4952228315222,-1.20497561405085,0.201799837144789));
#9811=CARTESIAN_POINT('Ctrl Pts',(10.4851784461209,-1.19439840869387,0.403646887802288));
#9812=CARTESIAN_POINT('Ctrl Pts',(10.4751339353761,-1.18382121389426,0.605493932788863));
#9813=CARTESIAN_POINT('Ctrl Pts',(10.4035069533234,-1.22105168617584,-3.13467776074076E-5));
#9814=CARTESIAN_POINT('Ctrl Pts',(10.3936624949941,-1.21047444506522,0.201815739766394));
#9815=CARTESIAN_POINT('Ctrl Pts',(10.3838179147697,-1.19989721405033,0.403662820908308));
#9816=CARTESIAN_POINT('Ctrl Pts',(10.3739732104882,-1.18931999337004,0.605509896555428));
#9817=CARTESIAN_POINT('Ctrl Pts',(10.3017512542637,-1.22646400658821,-1.55943981238903E-5));
#9818=CARTESIAN_POINT('Ctrl Pts',(10.2921066085356,-1.21588673949083,0.201831522212972));
#9819=CARTESIAN_POINT('Ctrl Pts',(10.2824618422276,-1.20530948226626,0.403678633593635));
#9820=CARTESIAN_POINT('Ctrl Pts',(10.2728169532007,-1.19473223514815,0.605525739654126));
#9821=CARTESIAN_POINT('Ctrl Pts',(10.2,-1.23178301601145,-4.5102810375397E-17));
#9822=CARTESIAN_POINT('Ctrl Pts',(10.1905551755811,-1.22120572247414,0.20184714636246));
#9823=CARTESIAN_POINT('Ctrl Pts',(10.1811102319487,-1.21062843858304,0.403694287664275));
#9824=CARTESIAN_POINT('Ctrl Pts',(10.1716651669877,-1.20005116456574,0.605541423818621));
#9825=CARTESIAN_POINT('',(10.4735630903435,-1.18390659316268,0.605494180667944));
#9826=CARTESIAN_POINT('Ctrl Pts',(10.1999999975038,-1.19856231440453,0.605472757505366));
#9827=CARTESIAN_POINT('Ctrl Pts',(10.2911933328565,-1.19375025772558,0.605479840815741));
#9828=CARTESIAN_POINT('Ctrl Pts',(10.3823809652617,-1.18886335120032,0.605486986548286));
#9829=CARTESIAN_POINT('Ctrl Pts',(10.4735630903435,-1.18390659316268,0.605494180667944));
#9830=CARTESIAN_POINT('Ctrl Pts',(10.4735630903435,-1.18390659316268,0.605494180667945));
#9831=CARTESIAN_POINT('Ctrl Pts',(10.4841302498201,-1.19445434834508,0.403662775875149));
#9832=CARTESIAN_POINT('Ctrl Pts',(10.4946974680575,-1.20500226999407,0.201831382381129));
#9833=CARTESIAN_POINT('Ctrl Pts',(10.5052647440597,-1.21555035534119,-6.86299975183324E-17));
#9834=CARTESIAN_POINT('Ctrl Pts',(10.,-1.10900986674273,0.7));
#9835=CARTESIAN_POINT('Ctrl Pts',(9.09944331332257,-1.15544418981837,0.7));
#9836=CARTESIAN_POINT('Ctrl Pts',(8.1984670949788,-1.19422430779862,0.7));
#9837=CARTESIAN_POINT('Ctrl Pts',(7.29709043526679,-1.22049830417059,0.7));
#9838=CARTESIAN_POINT('Ctrl Pts',(10.0014871213396,-1.13785139984992,0.7));
#9839=CARTESIAN_POINT('Ctrl Pts',(9.10076698492608,-1.18430758604571,0.700000491839571));
#9840=CARTESIAN_POINT('Ctrl Pts',(8.19957769811723,-1.22310890030201,0.699999704549177));
#9841=CARTESIAN_POINT('Ctrl Pts',(7.29793284700475,-1.24939875264889,0.7));
#9842=CARTESIAN_POINT('Ctrl Pts',(10.0040646682326,-1.18784086746588,0.676686753673613));
#9843=CARTESIAN_POINT('Ctrl Pts',(9.10306300621911,-1.23433322993607,0.676664155483858));
#9844=CARTESIAN_POINT('Ctrl Pts',(8.20149954052229,-1.27317186922949,0.676644146017133));
#9845=CARTESIAN_POINT('Ctrl Pts',(7.29939288958795,-1.29948813715084,0.676630595533454));
#9846=CARTESIAN_POINT('Ctrl Pts',(10.0050807923581,-1.20754778500352,0.627085325222079));
#9847=CARTESIAN_POINT('Ctrl Pts',(9.10396596140607,-1.25402923300358,0.627026849623412));
#9848=CARTESIAN_POINT('Ctrl Pts',(8.20225661204673,-1.29285896783792,0.626974637782525));
#9849=CARTESIAN_POINT('Ctrl Pts',(7.29996660609514,-1.31917051289423,0.626939603849942));
#9850=CARTESIAN_POINT('Ctrl Pts',(10.0051416645797,-1.20872835322339,0.605457722909465));
#9851=CARTESIAN_POINT('Ctrl Pts',(9.1040197884667,-1.25519559703033,0.605388684776982));
#9852=CARTESIAN_POINT('Ctrl Pts',(8.20230020786566,-1.29401302889245,0.605326714446839));
#9853=CARTESIAN_POINT('Ctrl Pts',(7.29999999953094,-1.32031613471704,0.605285370449856));
#9854=CARTESIAN_POINT('Ctrl Pts',(10.4681436286308,-1.08420482079362,0.7));
#9855=CARTESIAN_POINT('Ctrl Pts',(10.3770124662346,-1.0891584122264,0.7));
#9856=CARTESIAN_POINT('Ctrl Pts',(10.285877616441,-1.09404209584202,0.7));
#9857=CARTESIAN_POINT('Ctrl Pts',(10.1947388861048,-1.09885088260188,0.7));
#9858=CARTESIAN_POINT('Ctrl Pts',(10.4697107510168,-1.11303515260326,0.7));
#9859=CARTESIAN_POINT('Ctrl Pts',(10.3785648662465,-1.11799094453753,0.700000051218742));
#9860=CARTESIAN_POINT('Ctrl Pts',(10.2874149314686,-1.12287675076168,0.699999949550842));
#9861=CARTESIAN_POINT('Ctrl Pts',(10.196260416419,-1.12768774893097,0.7));
#9862=CARTESIAN_POINT('Ctrl Pts',(10.4724269697127,-1.16300539549315,0.676698381019543));
#9863=CARTESIAN_POINT('Ctrl Pts',(10.3812557252598,-1.16796482352885,0.676696026813929));
#9864=CARTESIAN_POINT('Ctrl Pts',(10.2900793016129,-1.17285439035486,0.676693724638983));
#9865=CARTESIAN_POINT('Ctrl Pts',(10.1988975981852,-1.17766904563614,0.67669140632491));
#9866=CARTESIAN_POINT('Ctrl Pts',(10.4734985149421,-1.18271860027509,0.627116141711795));
#9867=CARTESIAN_POINT('Ctrl Pts',(10.382317043787,-1.18767684023183,0.627110048826767));
#9868=CARTESIAN_POINT('Ctrl Pts',(10.2911301919381,-1.19256517083271,0.627104033151799));
#9869=CARTESIAN_POINT('Ctrl Pts',(10.1999375452555,-1.19737868557977,0.627098033786781));
#9870=CARTESIAN_POINT('Ctrl Pts',(10.4735630903435,-1.18390659316268,0.605494180667944));
#9871=CARTESIAN_POINT('Ctrl Pts',(10.3823809652617,-1.18886335120032,0.605486986548286));
#9872=CARTESIAN_POINT('Ctrl Pts',(10.2911933328565,-1.19375025772558,0.605479840815741));
#9873=CARTESIAN_POINT('Ctrl Pts',(10.1999999975038,-1.19856231440453,0.605472757505366));
#9874=CARTESIAN_POINT('',(10.4681436258201,-1.08420482094639,0.7));
#9875=CARTESIAN_POINT('Ctrl Pts',(10.4681436258201,-1.0842048209464,0.7));
#9876=CARTESIAN_POINT('Ctrl Pts',(10.3787660248044,-1.08906309452597,0.7));
#9877=CARTESIAN_POINT('Ctrl Pts',(10.289384876933,-1.09385412476048,0.7));
#9878=CARTESIAN_POINT('Ctrl Pts',(10.1999999999973,-1.09857320510493,0.7));
#9879=CARTESIAN_POINT('Origin',(10.4681436286308,-1.08420482099672,0.6));
#9880=CARTESIAN_POINT('Origin',(5.4,-8.11656130105013E-18,0.7));
#9881=CARTESIAN_POINT('',(10.4681436286308,1.08420482109828,0.7));
#9882=CARTESIAN_POINT('Ctrl Pts',(10.1999999980461,1.09857320520795,0.7));
#9883=CARTESIAN_POINT('Ctrl Pts',(10.2893848765692,1.09385412478074,0.7));
#9884=CARTESIAN_POINT('Ctrl Pts',(10.3787660260279,1.08906309446088,0.7));
#9885=CARTESIAN_POINT('Ctrl Pts',(10.4681436286308,1.08420482079361,0.7));
#9886=CARTESIAN_POINT('',(10.4681436286308,0.7,0.7));
#9887=CARTESIAN_POINT('Ctrl Pts',(7.3,1.35236351479305,-3.57463069561303E-11));
#9888=CARTESIAN_POINT('Ctrl Pts',(7.29625341766908,1.34178092325856,0.20193409200674));
#9889=CARTESIAN_POINT('Ctrl Pts',(7.29250676907475,1.33119833465113,0.403868182976914));
#9890=CARTESIAN_POINT('Ctrl Pts',(7.28876005303626,1.32061574904014,0.60580227285657));
#9891=CARTESIAN_POINT('Ctrl Pts',(8.20875307682014,1.32613868191819,-8.19770140467192E-5));
#9892=CARTESIAN_POINT('Ctrl Pts',(8.20321812688841,1.31555630757352,0.201851960063995));
#9893=CARTESIAN_POINT('Ctrl Pts',(8.19768309032092,1.3049739355521,0.403785895138154));
#9894=CARTESIAN_POINT('Ctrl Pts',(8.19214796413082,1.29439157094932,0.605719828284144));
#9895=CARTESIAN_POINT('Ctrl Pts',(9.11786336174626,1.28732002675385,-0.000205293251048056));
#9896=CARTESIAN_POINT('Ctrl Pts',(9.11054075262572,1.27673792860073,0.201728409716354));
#9897=CARTESIAN_POINT('Ctrl Pts',(9.10321803982063,1.26615583517412,0.403662109357089));
#9898=CARTESIAN_POINT('Ctrl Pts',(9.09589522044026,1.25557375159787,0.605595805709147));
#9899=CARTESIAN_POINT('Ctrl Pts',(10.0273290644402,1.2407389515511,-0.000342977407187712));
#9900=CARTESIAN_POINT('Ctrl Pts',(10.0182194939295,1.23015709330624,0.201590462897949));
#9901=CARTESIAN_POINT('Ctrl Pts',(10.0091098064748,1.21957524432641,0.403523898424684));
#9902=CARTESIAN_POINT('Ctrl Pts',(10.,1.20899340483035,0.605457329091028));
#9903=CARTESIAN_POINT('Ctrl Pts',(10.2,1.23178301601276,-2.39624899783797E-11));
#9904=CARTESIAN_POINT('Ctrl Pts',(10.1905551755807,1.22120572247504,0.201847146346486));
#9905=CARTESIAN_POINT('Ctrl Pts',(10.1811102319479,1.21062843858352,0.403694287656288));
#9906=CARTESIAN_POINT('Ctrl Pts',(10.1716651669865,1.2000511645658,0.605541423818621));
#9907=CARTESIAN_POINT('Ctrl Pts',(10.3017512542641,1.22646400658951,-1.55944220863836E-5));
#9908=CARTESIAN_POINT('Ctrl Pts',(10.2921066085356,1.2158867394917,0.201831522196997));
#9909=CARTESIAN_POINT('Ctrl Pts',(10.2824618422272,1.20530948226672,0.403678633585648));
#9910=CARTESIAN_POINT('Ctrl Pts',(10.2728169531999,1.19473223514819,0.605525739654127));
#9911=CARTESIAN_POINT('Ctrl Pts',(10.4035069533242,1.22105168617711,-3.13468015701665E-5));
#9912=CARTESIAN_POINT('Ctrl Pts',(10.3936624949945,1.21047444506608,0.201815739750419));
#9913=CARTESIAN_POINT('Ctrl Pts',(10.3838179147698,1.19989721405077,0.40366282090032));
#9914=CARTESIAN_POINT('Ctrl Pts',(10.3739732104878,1.18931999337006,0.605509896555428));
#9915=CARTESIAN_POINT('Ctrl Pts',(10.5052670937653,1.21555282972323,-4.72191118859062E-5));
#9916=CARTESIAN_POINT('Ctrl Pts',(10.495222831523,1.20497561405169,0.201799837128814));
#9917=CARTESIAN_POINT('Ctrl Pts',(10.4851784461213,1.19439840869429,0.403646887794301));
#9918=CARTESIAN_POINT('Ctrl Pts',(10.4751339353761,1.18382121389426,0.605493932788864));
#9919=CARTESIAN_POINT('',(10.4735630903435,1.18390659316268,0.605494180667944));
#9920=CARTESIAN_POINT('Ctrl Pts',(10.5052647440597,1.21555035534119,-4.0462425077159E-16));
#9921=CARTESIAN_POINT('Ctrl Pts',(10.4946974680575,1.20500226999407,0.201831382381129));
#9922=CARTESIAN_POINT('Ctrl Pts',(10.4841302498201,1.19445434834508,0.40366277587515));
#9923=CARTESIAN_POINT('Ctrl Pts',(10.4735630903435,1.18390659316268,0.605494180667945));
#9924=CARTESIAN_POINT('Ctrl Pts',(10.4735630903435,1.18390659316268,0.605494180667944));
#9925=CARTESIAN_POINT('Ctrl Pts',(10.3823809652617,1.18886335120032,0.605486986548286));
#9926=CARTESIAN_POINT('Ctrl Pts',(10.2911933328565,1.19375025772558,0.605479840815741));
#9927=CARTESIAN_POINT('Ctrl Pts',(10.1999999975038,1.19856231440453,0.605472757505366));
#9928=CARTESIAN_POINT('Origin',(7.1,1.42555555555556,0.));
#9929=CARTESIAN_POINT('',(7.0999999994629,-1.32593912634735,0.605276549957215));
#9930=CARTESIAN_POINT('Ctrl Pts',(7.0999999994629,-1.32593912634735,0.605276549957215));
#9931=CARTESIAN_POINT('Ctrl Pts',(7.0999999994629,-1.33126650931098,0.504490734647167));
#9932=CARTESIAN_POINT('Ctrl Pts',(7.1,-1.33659376385849,0.403703958452373));
#9933=CARTESIAN_POINT('Ctrl Pts',(7.1,-1.3472576786761,0.201945747207886));
#9934=CARTESIAN_POINT('Ctrl Pts',(7.1,-1.35259443928223,0.100972400854069));
#9935=CARTESIAN_POINT('Ctrl Pts',(7.1,-1.35793097395724,0.));
#9936=CARTESIAN_POINT('',(7.1,-1.22604182196417,0.7));
#9937=CARTESIAN_POINT('Ctrl Pts',(7.1,-1.22604182196307,0.7));
#9938=CARTESIAN_POINT('Ctrl Pts',(7.1,-1.23395163718705,0.7));
#9939=CARTESIAN_POINT('Ctrl Pts',(7.09999945440688,-1.24179783218049,0.699006056038995));
#9940=CARTESIAN_POINT('Ctrl Pts',(7.09999897931553,-1.2494401870438,0.697119011207626));
#9941=CARTESIAN_POINT('Ctrl Pts',(7.09999871186578,-1.25374240366384,0.696056710937424));
#9942=CARTESIAN_POINT('Ctrl Pts',(7.09999846845149,-1.25798007942473,0.69471034534287));
#9943=CARTESIAN_POINT('Ctrl Pts',(7.09999831430822,-1.26212651101681,0.6930909329195));
#9944=CARTESIAN_POINT('Ctrl Pts',(7.09999803835695,-1.26954956016987,0.690191818885951));
#9945=CARTESIAN_POINT('Ctrl Pts',(7.09999810102228,-1.27659977900265,0.686452252582521));
#9946=CARTESIAN_POINT('Ctrl Pts',(7.09999845706054,-1.28313109767173,0.681953977461377));
#9947=CARTESIAN_POINT('Ctrl Pts',(7.09999865314126,-1.2867280867584,0.679476645189077));
#9948=CARTESIAN_POINT('Ctrl Pts',(7.09999893113315,-1.29016742765117,0.67676830886676));
#9949=CARTESIAN_POINT('Ctrl Pts',(7.09999917787259,-1.2934208019838,0.673837071833988));
#9950=CARTESIAN_POINT('Ctrl Pts',(7.09999941835505,-1.29659167515528,0.670980166997299));
#9951=CARTESIAN_POINT('Ctrl Pts',(7.09999963169439,-1.29956664557352,0.667928795646746));
#9952=CARTESIAN_POINT('Ctrl Pts',(7.09999963110542,-1.30232317314677,0.664694459428825));
#9953=CARTESIAN_POINT('Ctrl Pts',(7.09999963001387,-1.30743194453681,0.658700148145236));
#9954=CARTESIAN_POINT('Ctrl Pts',(7.09999897381858,-1.31179333085743,0.652078782729069));
#9955=CARTESIAN_POINT('Ctrl Pts',(7.09999874753952,-1.31534789998199,0.64499600756552));
#9956=CARTESIAN_POINT('Ctrl Pts',(7.09999872438549,-1.31571162172319,0.644271261689237));
#9957=CARTESIAN_POINT('Ctrl Pts',(7.0999987046402,-1.31606685549941,0.643541664816448));
#9958=CARTESIAN_POINT('Ctrl Pts',(7.09999868869212,-1.31641350913238,0.642807383257706));
#9959=CARTESIAN_POINT('Ctrl Pts',(7.09999853283271,-1.31980133087414,0.635631300872562));
#9960=CARTESIAN_POINT('Ctrl Pts',(7.09999885939544,-1.32233451509485,0.628092322434426));
#9961=CARTESIAN_POINT('Ctrl Pts',(7.09999934101855,-1.32395982399511,0.620358959365968));
#9962=CARTESIAN_POINT('Ctrl Pts',(7.09999964997549,-1.32500244522074,0.615398075635307));
#9963=CARTESIAN_POINT('Ctrl Pts',(7.09999999934316,-1.32567060646853,0.610356529630438));
#9964=CARTESIAN_POINT('Ctrl Pts',(7.09999999981141,-1.32593912630714,0.60527654995744));
#9965=CARTESIAN_POINT('',(7.09999999995537,1.22604182196549,0.7));
#9966=CARTESIAN_POINT('',(7.1,0.712777777777778,0.7));
#9967=CARTESIAN_POINT('',(7.0999999994629,1.32593912634735,0.605276549957215));
#9968=CARTESIAN_POINT('Ctrl Pts',(7.09999999981142,1.32593912630714,0.60527654995744));
#9969=CARTESIAN_POINT('Ctrl Pts',(7.09999999908198,1.32552083177145,0.613190035045322));
#9970=CARTESIAN_POINT('Ctrl Pts',(7.09999922367565,1.32413525001942,0.621012727860624));
#9971=CARTESIAN_POINT('Ctrl Pts',(7.09999888117586,1.32186630199077,0.628584136488803));
#9972=CARTESIAN_POINT('Ctrl Pts',(7.09999868987568,1.32059900146923,0.632813078704371));
#9973=CARTESIAN_POINT('Ctrl Pts',(7.09999860640034,1.3190551184949,0.636963663611311));
#9974=CARTESIAN_POINT('Ctrl Pts',(7.09999865766138,1.31724253497577,0.641005923298765));
#9975=CARTESIAN_POINT('Ctrl Pts',(7.0999987494091,1.31399834762864,0.648240816253195));
#9976=CARTESIAN_POINT('Ctrl Pts',(7.09999933613984,1.30993159792479,0.655050690394837));
#9977=CARTESIAN_POINT('Ctrl Pts',(7.09999956222935,1.30510592187917,0.661272231165006));
#9978=CARTESIAN_POINT('Ctrl Pts',(7.09999960444598,1.30420484616769,0.662433950108221));
#9979=CARTESIAN_POINT('Ctrl Pts',(7.09999963060969,1.30327718139331,0.663575086117144));
#9980=CARTESIAN_POINT('Ctrl Pts',(7.09999963056866,1.30232317316131,0.664694459428815));
#9981=CARTESIAN_POINT('Ctrl Pts',(7.09999963048683,1.30042028596585,0.666927187690779));
#9982=CARTESIAN_POINT('Ctrl Pts',(7.09999952705857,1.29841262431024,0.669073382394206));
#9983=CARTESIAN_POINT('Ctrl Pts',(7.09999938633452,1.29630755303174,0.671129253595323));
#9984=CARTESIAN_POINT('Ctrl Pts',(7.09999900634735,1.29062337821964,0.676680576924663));
#9985=CARTESIAN_POINT('Ctrl Pts',(7.09999841760642,1.2842958957007,0.681513596217188));
#9986=CARTESIAN_POINT('Ctrl Pts',(7.0999982224057,1.2774887935492,0.68557385059291));
#9987=CARTESIAN_POINT('Ctrl Pts',(7.09999809840912,1.27316474526651,0.688153029745784));
#9988=CARTESIAN_POINT('Ctrl Pts',(7.09999810738417,1.26864620899217,0.690419707112974));
#9989=CARTESIAN_POINT('Ctrl Pts',(7.09999825155258,1.26396949224645,0.69235064530212));
#9990=CARTESIAN_POINT('Ctrl Pts',(7.09999847710269,1.25665281355793,0.695371579659609));
#9991=CARTESIAN_POINT('Ctrl Pts',(7.09999903441007,1.2490339950321,0.697538299034574));
#9992=CARTESIAN_POINT('Ctrl Pts',(7.09999948258254,1.24125996729125,0.698781081437474));
#9993=CARTESIAN_POINT('Ctrl Pts',(7.09999977198436,1.23623998534067,0.699583592753232));
#9994=CARTESIAN_POINT('Ctrl Pts',(7.1,1.23115469319345,0.7));
#9995=CARTESIAN_POINT('Ctrl Pts',(7.1,1.22604182196307,0.7));
#9996=CARTESIAN_POINT('Ctrl Pts',(7.1,1.35793097395724,0.));
#9997=CARTESIAN_POINT('Ctrl Pts',(7.1,1.35259441576718,0.100972845781549));
#9998=CARTESIAN_POINT('Ctrl Pts',(7.1,1.34725763161617,0.201946637598055));
#9999=CARTESIAN_POINT('Ctrl Pts',(7.1,1.33659371676552,0.403704849408333));
#10000=CARTESIAN_POINT('Ctrl Pts',(7.0999999994629,1.33126648576411,0.504491180117376));
#10001=CARTESIAN_POINT('Ctrl Pts',(7.0999999994629,1.32593912634735,0.605276549957215));
#10002=CARTESIAN_POINT('Ctrl Pts',(7.11011156210589,-1.35766432821499,-9.27062925672982E-5));
#10003=CARTESIAN_POINT('Ctrl Pts',(7.10674110347764,-1.34708925835705,0.201697046690488));
#10004=CARTESIAN_POINT('Ctrl Pts',(7.10337058314201,-1.33651419103807,0.403486798779133));
#10005=CARTESIAN_POINT('Ctrl Pts',(7.09999999999996,-1.32593912631822,0.605276549958221));
#10006=CARTESIAN_POINT('Ctrl Pts',(5.9694837631095,-1.38835096090528,2.80675674898241E-6));
#10007=CARTESIAN_POINT('Ctrl Pts',(5.96835662351021,-1.37777563343505,0.201792740207853));
#10008=CARTESIAN_POINT('Ctrl Pts',(5.96722945517891,-1.3672003004237,0.40358267322573));
#10009=CARTESIAN_POINT('Ctrl Pts',(5.96610224583462,-1.35662497356325,0.605372606931572));
#10010=CARTESIAN_POINT('Ctrl Pts',(4.8294200007394,-1.39866452387306,3.01102374082134E-5));
#10011=CARTESIAN_POINT('Ctrl Pts',(4.83053730380309,-1.38808904115766,0.201820093264151));
#10012=CARTESIAN_POINT('Ctrl Pts',(4.83165461298617,-1.3775135517806,0.403610075973038));
#10013=CARTESIAN_POINT('Ctrl Pts',(4.83277191472125,-1.36693806692183,0.605400059795761));
#10014=CARTESIAN_POINT('Ctrl Pts',(3.68991216363982,-1.37907703205181,-6.2684699445455E-5));
#10015=CARTESIAN_POINT('Ctrl Pts',(3.69327498756969,-1.36850179198701,0.201727122618256));
#10016=CARTESIAN_POINT('Ctrl Pts',(3.69663785098144,-1.3579265529724,0.403516929334346));
#10017=CARTESIAN_POINT('Ctrl Pts',(3.70000075457889,-1.34735131503281,0.605306735438421));
#10018=CARTESIAN_POINT('Ctrl Pts',(3.69999999992215,-1.34735368792773,0.6052614572053));
#10019=CARTESIAN_POINT('Ctrl Pts',(4.83355316856959,-1.366961322855,0.605214762857233));
#10020=CARTESIAN_POINT('Ctrl Pts',(5.96724522208681,-1.35660163688233,0.605228569880684));
#10021=CARTESIAN_POINT('Ctrl Pts',(7.09999999927392,-1.32593912632169,0.605276549957417));
#10022=CARTESIAN_POINT('Ctrl Pts',(7.1,-1.22604182196307,0.7));
#10023=CARTESIAN_POINT('Ctrl Pts',(5.96696284938742,-1.25674179781664,0.7));
#10024=CARTESIAN_POINT('Ctrl Pts',(4.83327074934872,-1.26710800714677,0.7));
#10025=CARTESIAN_POINT('Ctrl Pts',(3.7,-1.24747724070879,0.7));
#10026=CARTESIAN_POINT('Ctrl Pts',(7.10078315634008,-1.25494559805327,0.7));
#10027=CARTESIAN_POINT('Ctrl Pts',(5.96739926106349,-1.28566432005869,0.700000343763215));
#10028=CARTESIAN_POINT('Ctrl Pts',(4.83328164159484,-1.29603890521481,0.700000334703603));
#10029=CARTESIAN_POINT('Ctrl Pts',(3.69949916377151,-1.27639017438114,0.7));
#10030=CARTESIAN_POINT('Ctrl Pts',(7.10214055788579,-1.30504291366416,0.676629771601708));
#10031=CARTESIAN_POINT('Ctrl Pts',(5.96815960929481,-1.33579288254824,0.676614006760374));
#10032=CARTESIAN_POINT('Ctrl Pts',(4.83329467960724,-1.3461818279488,0.676609489640654));
#10033=CARTESIAN_POINT('Ctrl Pts',(3.69863109538965,-1.3265031696486,0.676624836591801));
#10034=CARTESIAN_POINT('Ctrl Pts',(7.10267376869946,-1.32472200604796,0.626932241521275));
#10035=CARTESIAN_POINT('Ctrl Pts',(5.9684558952243,-1.35546668061705,0.626891484245174));
#10036=CARTESIAN_POINT('Ctrl Pts',(4.83330292199863,-1.36585610284781,0.626879766983475));
#10037=CARTESIAN_POINT('Ctrl Pts',(3.69829020046733,-1.34618280086838,0.626919440930842));
#10038=CARTESIAN_POINT('Ctrl Pts',(7.10270476209941,-1.32586587253612,0.605276664588022));
#10039=CARTESIAN_POINT('Ctrl Pts',(5.96847377630401,-1.35660073810322,0.605228567467576));
#10040=CARTESIAN_POINT('Ctrl Pts',(4.8333022084086,-1.36698748587873,0.605214711607465));
#10041=CARTESIAN_POINT('Ctrl Pts',(3.69827043673666,-1.34732374755196,0.60526152849799));
#10042=CARTESIAN_POINT('Ctrl Pts',(7.1,-1.22604182196307,0.7));
#10043=CARTESIAN_POINT('Ctrl Pts',(5.96696284938742,-1.25674179781664,0.7));
#10044=CARTESIAN_POINT('Ctrl Pts',(4.83327074934872,-1.26710800714677,0.7));
#10045=CARTESIAN_POINT('Ctrl Pts',(3.7,-1.24747724070879,0.7));
#10046=CARTESIAN_POINT('Origin',(5.4,-8.11656130105013E-18,0.7));
#10047=CARTESIAN_POINT('Ctrl Pts',(3.7,1.24747724070879,0.7));
#10048=CARTESIAN_POINT('Ctrl Pts',(4.83327074934871,1.26710800714677,0.7));
#10049=CARTESIAN_POINT('Ctrl Pts',(5.96696284938742,1.25674179781664,0.7));
#10050=CARTESIAN_POINT('Ctrl Pts',(7.1,1.22604182196307,0.7));
#10051=CARTESIAN_POINT('Ctrl Pts',(3.7,1.24747724070879,0.7));
#10052=CARTESIAN_POINT('Ctrl Pts',(4.83327074934871,1.26710800714677,0.7));
#10053=CARTESIAN_POINT('Ctrl Pts',(5.96696284938742,1.25674179781664,0.7));
#10054=CARTESIAN_POINT('Ctrl Pts',(7.1,1.22604182196307,0.7));
#10055=CARTESIAN_POINT('Ctrl Pts',(3.69949916377151,1.27639017438114,0.7));
#10056=CARTESIAN_POINT('Ctrl Pts',(4.83328164159484,1.29603890521481,0.700000334703603));
#10057=CARTESIAN_POINT('Ctrl Pts',(5.96739926106349,1.28566432005869,0.700000343763215));
#10058=CARTESIAN_POINT('Ctrl Pts',(7.10078315634008,1.25494559805327,0.7));
#10059=CARTESIAN_POINT('Ctrl Pts',(3.69863109538965,1.3265031696486,0.676624836591801));
#10060=CARTESIAN_POINT('Ctrl Pts',(4.83329467960724,1.3461818279488,0.676609489640654));
#10061=CARTESIAN_POINT('Ctrl Pts',(5.9681596092948,1.33579288254824,0.676614006760374));
#10062=CARTESIAN_POINT('Ctrl Pts',(7.10214055788579,1.30504291366416,0.676629771601707));
#10063=CARTESIAN_POINT('Ctrl Pts',(3.69829020046733,1.34618280086838,0.626919440930842));
#10064=CARTESIAN_POINT('Ctrl Pts',(4.83330292199863,1.36585610284781,0.626879766983475));
#10065=CARTESIAN_POINT('Ctrl Pts',(5.9684558952243,1.35546668061705,0.626891484245174));
#10066=CARTESIAN_POINT('Ctrl Pts',(7.10267376869946,1.32472200604796,0.626932241521275));
#10067=CARTESIAN_POINT('Ctrl Pts',(3.69827043673666,1.34732374755196,0.60526152849799));
#10068=CARTESIAN_POINT('Ctrl Pts',(4.83330220840859,1.36698748587873,0.605214711607465));
#10069=CARTESIAN_POINT('Ctrl Pts',(5.96847377630401,1.35660073810322,0.605228567467576));
#10070=CARTESIAN_POINT('Ctrl Pts',(7.10270476209941,1.32586587253612,0.605276664588022));
#10071=CARTESIAN_POINT('Ctrl Pts',(7.09999999927392,1.32593912632169,0.605276549957417));
#10072=CARTESIAN_POINT('Ctrl Pts',(5.96724522208681,1.35660163688233,0.605228569880684));
#10073=CARTESIAN_POINT('Ctrl Pts',(4.83355316856959,1.366961322855,0.605214762857233));
#10074=CARTESIAN_POINT('Ctrl Pts',(3.69999999992215,1.34735368792773,0.6052614572053));
#10075=CARTESIAN_POINT('Ctrl Pts',(3.68991216360307,1.37907703216746,-6.26869063400631E-5));
#10076=CARTESIAN_POINT('Ctrl Pts',(3.6932749875452,1.36850179206412,0.201727121146993));
#10077=CARTESIAN_POINT('Ctrl Pts',(3.69663785096921,1.35792655301095,0.403516928598715));
#10078=CARTESIAN_POINT('Ctrl Pts',(3.70000075457892,1.34735131503281,0.605306735438421));
#10079=CARTESIAN_POINT('Ctrl Pts',(4.8294200007272,1.39866452398872,3.01080305115927E-5));
#10080=CARTESIAN_POINT('Ctrl Pts',(4.83053730379496,1.38808904123477,0.201820091792887));
#10081=CARTESIAN_POINT('Ctrl Pts',(4.83165461298211,1.37751355181915,0.403610075237406));
#10082=CARTESIAN_POINT('Ctrl Pts',(4.83277191472127,1.36693806692183,0.605400059795761));
#10083=CARTESIAN_POINT('Ctrl Pts',(5.96948376312183,1.38835096102094,2.80454985295556E-6));
#10084=CARTESIAN_POINT('Ctrl Pts',(5.96835662351844,1.37777563351215,0.201792738736588));
#10085=CARTESIAN_POINT('Ctrl Pts',(5.96722945518303,1.36720030046225,0.403582672490098));
#10086=CARTESIAN_POINT('Ctrl Pts',(5.96610224583462,1.35662497356325,0.605372606931572));
#10087=CARTESIAN_POINT('Ctrl Pts',(7.11011156214274,1.35766432833065,-9.27084994613511E-5));
#10088=CARTESIAN_POINT('Ctrl Pts',(7.10674110350221,1.34708925843416,0.201697045219225));
#10089=CARTESIAN_POINT('Ctrl Pts',(7.10337058315429,1.33651419107662,0.403486798043502));
#10090=CARTESIAN_POINT('Ctrl Pts',(7.09999999999996,1.32593912631822,0.605276549958221));
#10091=CARTESIAN_POINT('Origin',(3.5,1.44777777777778,0.));
#10092=CARTESIAN_POINT('',(3.5,-1.34358136363184,0.605270327458634));
#10093=CARTESIAN_POINT('Ctrl Pts',(3.5,-1.34358136363184,0.605270327458634));
#10094=CARTESIAN_POINT('Ctrl Pts',(3.5,-1.34890136370362,0.504489156176152));
#10095=CARTESIAN_POINT('Ctrl Pts',(3.5,-1.35422123464986,0.403706701640381));
#10096=CARTESIAN_POINT('Ctrl Pts',(3.5,-1.3648706701715,0.201950780690867));
#10097=CARTESIAN_POINT('Ctrl Pts',(3.5,-1.3702003690246,0.100974756199658));
#10098=CARTESIAN_POINT('Ctrl Pts',(3.5,-1.37552980833516,0.));
#10099=CARTESIAN_POINT('',(3.5,-1.24369946473884,0.7));
#10100=CARTESIAN_POINT('Ctrl Pts',(3.49999999991873,-1.24369946470729,0.7));
#10101=CARTESIAN_POINT('Ctrl Pts',(3.49999999896975,-1.25160831520001,0.699999999810925));
#10102=CARTESIAN_POINT('Ctrl Pts',(3.50000040534574,-1.25945374057332,0.69900619751828));
#10103=CARTESIAN_POINT('Ctrl Pts',(3.50000075715473,-1.26709539726361,0.697119355224275));
#10104=CARTESIAN_POINT('Ctrl Pts',(3.5000009551612,-1.27139630362835,0.696057395447694));
#10105=CARTESIAN_POINT('Ctrl Pts',(3.50000113454144,-1.27563271975905,0.694711510656402));
#10106=CARTESIAN_POINT('Ctrl Pts',(3.50000124621709,-1.27977793997275,0.693092697679401));
#10107=CARTESIAN_POINT('Ctrl Pts',(3.50000144618968,-1.28720060051191,0.690193961644836));
#10108=CARTESIAN_POINT('Ctrl Pts',(3.50000138985083,-1.29425038514255,0.686454755369034));
#10109=CARTESIAN_POINT('Ctrl Pts',(3.5000011147959,-1.30078112659466,0.681956784255818));
#10110=CARTESIAN_POINT('Ctrl Pts',(3.50000096334461,-1.30437709646577,0.679480102439082));
#10111=CARTESIAN_POINT('Ctrl Pts',(3.50000075087427,-1.30781543681835,0.676772489296601));
#10112=CARTESIAN_POINT('Ctrl Pts',(3.50000056308077,-1.31106783354026,0.67384203444854));
#10113=CARTESIAN_POINT('Ctrl Pts',(3.50000037990614,-1.31424023611357,0.670983655445047));
#10114=CARTESIAN_POINT('Ctrl Pts',(3.50000021841608,-1.31721646102264,0.667930553458483));
#10115=CARTESIAN_POINT('Ctrl Pts',(3.50000022028926,-1.3199739184757,0.664694242102541));
#10116=CARTESIAN_POINT('Ctrl Pts',(3.50000022375892,-1.32508151834405,0.658699667848218));
#10117=CARTESIAN_POINT('Ctrl Pts',(3.50000072745304,-1.32944146850927,0.652077914129702));
#10118=CARTESIAN_POINT('Ctrl Pts',(3.50000090782832,-1.33299465793893,0.64499486611401));
#10119=CARTESIAN_POINT('Ctrl Pts',(3.50000092626355,-1.33335781125732,0.644270944003422));
#10120=CARTESIAN_POINT('Ctrl Pts',(3.50000094214549,-1.33371249714824,0.643542183465449));
#10121=CARTESIAN_POINT('Ctrl Pts',(3.5000009551778,-1.33405862411533,0.642808750463418));
#10122=CARTESIAN_POINT('Ctrl Pts',(3.50000108270827,-1.3374457225345,0.635631587173848));
#10123=CARTESIAN_POINT('Ctrl Pts',(3.5000008470667,-1.33997810357527,0.628091493562486));
#10124=CARTESIAN_POINT('Ctrl Pts',(3.50000049017339,-1.34160279315579,0.620357239364781));
#10125=CARTESIAN_POINT('Ctrl Pts',(3.50000026118253,-1.3426452308862,0.615394766232079));
#10126=CARTESIAN_POINT('Ctrl Pts',(3.5,-1.34331313055125,0.610351689051435));
#10127=CARTESIAN_POINT('Ctrl Pts',(3.5,-1.34358136363184,0.605270327458634));
#10128=CARTESIAN_POINT('',(3.5,0.723888888888889,0.7));
#10129=CARTESIAN_POINT('Ctrl Pts',(3.5,1.37552980833516,0.));
#10130=CARTESIAN_POINT('Ctrl Pts',(3.5,1.37020035376703,0.10097504527886));
#10131=CARTESIAN_POINT('Ctrl Pts',(3.5,1.36487063968137,0.201951358354439));
#10132=CARTESIAN_POINT('Ctrl Pts',(3.5,1.35422120417274,0.403707279015233));
#10133=CARTESIAN_POINT('Ctrl Pts',(3.5,1.34890134846466,0.504489444860456));
#10134=CARTESIAN_POINT('Ctrl Pts',(3.5,1.34358136363184,0.605270327458635));
#10135=CARTESIAN_POINT('Ctrl Pts',(3.50000000097418,-1.37552980835478,3.46944695195361E-18));
#10136=CARTESIAN_POINT('Ctrl Pts',(3.50374047168104,-1.36494504174376,0.201972406882836));
#10137=CARTESIAN_POINT('Ctrl Pts',(3.50748098869546,-1.35436027657305,0.403944812985359));
#10138=CARTESIAN_POINT('Ctrl Pts',(3.51122155284351,-1.34377551287676,0.605917218294091));
#10139=CARTESIAN_POINT('Ctrl Pts',(2.69119625874569,-1.35924722858667,-7.54309614812119E-5));
#10140=CARTESIAN_POINT('Ctrl Pts',(2.69653217397324,-1.34866266892899,0.20189683354744));
#10141=CARTESIAN_POINT('Ctrl Pts',(2.70186816749714,-1.3380781117335,0.403869096002786));
#10142=CARTESIAN_POINT('Ctrl Pts',(2.7072042346663,-1.32749355863083,0.605841357314298));
#10143=CARTESIAN_POINT('Ctrl Pts',(1.88267190563219,-1.32763345268679,-0.000212792412547521));
#10144=CARTESIAN_POINT('Ctrl Pts',(1.88960380459144,-1.31704931403188,0.201759213581099));
#10145=CARTESIAN_POINT('Ctrl Pts',(1.89653581411498,-1.30646518166523,0.403731216009517));
#10146=CARTESIAN_POINT('Ctrl Pts',(1.90346792975642,-1.29588105699583,0.605703215867581));
#10147=CARTESIAN_POINT('Ctrl Pts',(1.07441451989529,-1.27728918272486,-0.000429194541766893));
#10148=CARTESIAN_POINT('Ctrl Pts',(1.08294287068452,-1.26670581246828,0.201542410257184));
#10149=CARTESIAN_POINT('Ctrl Pts',(1.09147136321593,-1.25612245578053,0.403514009799157));
#10150=CARTESIAN_POINT('Ctrl Pts',(1.09999999999989,-1.24553911298205,0.605485603995245));
#10151=CARTESIAN_POINT('Ctrl Pts',(1.09999999916631,-1.24553911263844,0.605485603997431));
#10152=CARTESIAN_POINT('Ctrl Pts',(1.89930203168262,-1.29563783986497,0.605377360150118));
#10153=CARTESIAN_POINT('Ctrl Pts',(2.69958486793449,-1.32722445934619,0.605308375488923));
#10154=CARTESIAN_POINT('Ctrl Pts',(3.5,-1.34358136363184,0.605270327458634));
#10155=CARTESIAN_POINT('Ctrl Pts',(3.50204003610941,-1.24374118183538,0.7));
#10156=CARTESIAN_POINT('Ctrl Pts',(2.70080437300401,-1.2273695200909,0.7));
#10157=CARTESIAN_POINT('Ctrl Pts',(1.89984199608574,-1.1957170361627,0.7));
#10158=CARTESIAN_POINT('Ctrl Pts',(1.1,-1.14549341399196,0.7));
#10159=CARTESIAN_POINT('Ctrl Pts',(3.50144932661635,-1.27265074030048,0.7));
#10160=CARTESIAN_POINT('Ctrl Pts',(2.6998452019678,-1.25626413437997,0.699999727319846));
#10161=CARTESIAN_POINT('Ctrl Pts',(1.89847848223078,-1.22458382597074,0.70000077422621));
#10162=CARTESIAN_POINT('Ctrl Pts',(1.09819048660397,-1.17431102498992,0.7));
#10163=CARTESIAN_POINT('Ctrl Pts',(3.50042536655637,-1.322763754511,0.676632802377821));
#10164=CARTESIAN_POINT('Ctrl Pts',(2.69818680938114,-1.3063522351595,0.67664530655333));
#10165=CARTESIAN_POINT('Ctrl Pts',(1.89610976425884,-1.27462253270773,0.67666760713801));
#10166=CARTESIAN_POINT('Ctrl Pts',(1.09505363188407,-1.22426736091617,0.676703190608825));
#10167=CARTESIAN_POINT('Ctrl Pts',(3.50002334924346,-1.34243864233338,0.626926882269943));
#10168=CARTESIAN_POINT('Ctrl Pts',(2.6975332861013,-1.32603127467068,0.626959208652505));
#10169=CARTESIAN_POINT('Ctrl Pts',(1.89518106151152,-1.29430885982199,0.62701751976321));
#10170=CARTESIAN_POINT('Ctrl Pts',(1.09381704710221,-1.24396073223232,0.627109609335854));
#10171=CARTESIAN_POINT('Ctrl Pts',(3.5,-1.34358136363184,0.605270327458634));
#10172=CARTESIAN_POINT('Ctrl Pts',(2.69749615303,-1.32718177535833,0.605308474776761));
#10173=CARTESIAN_POINT('Ctrl Pts',(1.89512529323683,-1.29547288309274,0.605377720397184));
#10174=CARTESIAN_POINT('Ctrl Pts',(1.09374258853658,-1.24514653057163,0.605486452199395));
#10175=CARTESIAN_POINT('Ctrl Pts',(3.49999999991875,-1.24369946470729,0.7));
#10176=CARTESIAN_POINT('Ctrl Pts',(3.26917843083003,-1.23897560807887,0.7));
#10177=CARTESIAN_POINT('Ctrl Pts',(3.03837960179139,-1.23298334389983,0.7));
#10178=CARTESIAN_POINT('Ctrl Pts',(2.80762376541487,-1.22564400623233,0.7));
#10179=CARTESIAN_POINT('Ctrl Pts',(2.57739190516312,-1.2178709162388,0.7));
#10180=CARTESIAN_POINT('Ctrl Pts',(2.08463535466707,-1.20026407570248,0.7));
#10181=CARTESIAN_POINT('Ctrl Pts',(1.59210562457525,-1.17639367564078,0.7));
#10182=CARTESIAN_POINT('Ctrl Pts',(1.1,-1.14549341399196,0.7));
#10183=CARTESIAN_POINT('Origin',(5.4,-8.11656130105013E-18,0.7));
#10184=CARTESIAN_POINT('Ctrl Pts',(1.0744145198953,1.27728918272486,-0.000429194541767127));
#10185=CARTESIAN_POINT('Ctrl Pts',(1.08294287068452,1.26670581246828,0.201542410257184));
#10186=CARTESIAN_POINT('Ctrl Pts',(1.09147136321593,1.25612245578053,0.403514009799157));
#10187=CARTESIAN_POINT('Ctrl Pts',(1.0999999999999,1.24553911298205,0.605485603995245));
#10188=CARTESIAN_POINT('Ctrl Pts',(1.88267190563235,1.3276334526868,-0.000212792412547728));
#10189=CARTESIAN_POINT('Ctrl Pts',(1.8896038045916,1.31704931403189,0.201759213581098));
#10190=CARTESIAN_POINT('Ctrl Pts',(1.89653581411514,1.30646518166524,0.403731216009517));
#10191=CARTESIAN_POINT('Ctrl Pts',(1.90346792975658,1.29588105699584,0.605703215867581));
#10192=CARTESIAN_POINT('Ctrl Pts',(2.69119625874601,1.35924722858668,-7.54309614812134E-5));
#10193=CARTESIAN_POINT('Ctrl Pts',(2.69653217397356,1.348662668929,0.201896833547441));
#10194=CARTESIAN_POINT('Ctrl Pts',(2.70186816749745,1.33807811173351,0.403869096002786));
#10195=CARTESIAN_POINT('Ctrl Pts',(2.70720423466661,1.32749355863085,0.605841357314298));
#10196=CARTESIAN_POINT('Ctrl Pts',(3.50000000097466,1.37552980835479,-3.81639164714898E-17));
#10197=CARTESIAN_POINT('Ctrl Pts',(3.50374047168151,1.36494504174377,0.201972406882836));
#10198=CARTESIAN_POINT('Ctrl Pts',(3.50748098869594,1.35436027657306,0.403944812985359));
#10199=CARTESIAN_POINT('Ctrl Pts',(3.51122155284398,1.34377551287677,0.605917218294091));
#10200=CARTESIAN_POINT('Origin',(0.9,1.34328341716202,0.));
#10201=CARTESIAN_POINT('',(0.9,-1.23261418131727,0.605513513251856));
#10202=CARTESIAN_POINT('Ctrl Pts',(0.9,-1.23261418131727,0.605513513251856));
#10203=CARTESIAN_POINT('Ctrl Pts',(0.9,-1.23820195798151,0.504544236118289));
#10204=CARTESIAN_POINT('Ctrl Pts',(0.9,-1.24378834611607,0.403573587101897));
#10205=CARTESIAN_POINT('Ctrl Pts',(0.9,-1.25495246062481,0.201736610752668));
#10206=CARTESIAN_POINT('Ctrl Pts',(0.9,-1.26053033259331,0.100867703930409));
#10207=CARTESIAN_POINT('Ctrl Pts',(0.9,-1.266106713614,0.));
#10208=CARTESIAN_POINT('',(0.9,-1.13254484134404,0.7));
#10209=CARTESIAN_POINT('Ctrl Pts',(0.899999999937205,-1.13254484130906,
0.7));
#10210=CARTESIAN_POINT('Ctrl Pts',(0.899999996287105,-1.14047016437301,
0.699999998205918));
#10211=CARTESIAN_POINT('Ctrl Pts',(0.900001280561548,-1.14833327216777,
0.699006663725481));
#10212=CARTESIAN_POINT('Ctrl Pts',(0.900002371513522,-1.15599299513142,
0.697119896446058));
#10213=CARTESIAN_POINT('Ctrl Pts',(0.900002982478546,-1.16028266409831,
0.696063251566776));
#10214=CARTESIAN_POINT('Ctrl Pts',(0.900003528700818,-1.16450859688491,
0.694725368779139));
#10215=CARTESIAN_POINT('Ctrl Pts',(0.900003857331964,-1.16864431737637,
0.693116947675672));
#10216=CARTESIAN_POINT('Ctrl Pts',(0.900004447924614,-1.17607674172948,
0.690226407030055));
#10217=CARTESIAN_POINT('Ctrl Pts',(0.900004211500339,-1.18313828052408,
0.686496282267003));
#10218=CARTESIAN_POINT('Ctrl Pts',(0.900003280035406,-1.18968205680082,
0.682006679400108));
#10219=CARTESIAN_POINT('Ctrl Pts',(0.900002768383153,-1.19327654302499,
0.679540547464272));
#10220=CARTESIAN_POINT('Ctrl Pts',(0.900002064672634,-1.19671453445753,
0.676844382327844));
#10221=CARTESIAN_POINT('Ctrl Pts',(0.900001450170085,-1.19996775918788,
0.673925988054463));
#10222=CARTESIAN_POINT('Ctrl Pts',(0.900000850201302,-1.20314404102283,
0.67107661751105));
#10223=CARTESIAN_POINT('Ctrl Pts',(0.900000329673364,-1.20612495630093,
0.668032594545539));
#10224=CARTESIAN_POINT('Ctrl Pts',(0.900000346081477,-1.20888784276431,
0.664805176146368));
#10225=CARTESIAN_POINT('Ctrl Pts',(0.900000376514472,-1.21401231436848,
0.658819112599938));
#10226=CARTESIAN_POINT('Ctrl Pts',(0.900002057232535,-1.21838968018573,
0.652203523053766));
#10227=CARTESIAN_POINT('Ctrl Pts',(0.900002698394847,-1.22195969054856,
0.645123732731769));
#10228=CARTESIAN_POINT('Ctrl Pts',(0.900002763240662,-1.22232075393107,
0.644407697543824));
#10229=CARTESIAN_POINT('Ctrl Pts',(0.90000282009371,-1.22267351953901,0.643686895083047));
#10230=CARTESIAN_POINT('Ctrl Pts',(0.900002868017411,-1.22301789747605,
0.642961485862499));
#10231=CARTESIAN_POINT('Ctrl Pts',(0.900003341628975,-1.22642125256928,
0.635792544708285));
#10232=CARTESIAN_POINT('Ctrl Pts',(0.900002645022176,-1.22896979279554,
0.628258742918086));
#10233=CARTESIAN_POINT('Ctrl Pts',(0.900001532827652,-1.23061007098772,
0.6205286650049));
#10234=CARTESIAN_POINT('Ctrl Pts',(0.900000822323555,-1.23165793118585,
0.61559045329652));
#10235=CARTESIAN_POINT('Ctrl Pts',(0.900000000000001,-1.23233426661673,
0.610571479357261));
#10236=CARTESIAN_POINT('Ctrl Pts',(0.900000000000001,-1.23261418131727,
0.605513513251856));
#10237=CARTESIAN_POINT('',(0.9,1.13254484134404,0.7));
#10238=CARTESIAN_POINT('',(0.9,0.671641708581009,0.7));
#10239=CARTESIAN_POINT('',(0.9,1.23261418131727,0.605513513251856));
#10240=CARTESIAN_POINT('Ctrl Pts',(0.9,1.23261418131727,0.605513513251856));
#10241=CARTESIAN_POINT('Ctrl Pts',(0.9,1.23217633603244,0.613425232807268));
#10242=CARTESIAN_POINT('Ctrl Pts',(0.900001832787994,1.23077105609892,0.621244170085157));
#10243=CARTESIAN_POINT('Ctrl Pts',(0.900002580745575,1.22848219166492,0.628809599741497));
#10244=CARTESIAN_POINT('Ctrl Pts',(0.900002993068559,1.22722042035689,0.632980157827643));
#10245=CARTESIAN_POINT('Ctrl Pts',(0.90000314174678,1.22568915198244,0.637073706995481));
#10246=CARTESIAN_POINT('Ctrl Pts',(0.900002971484041,1.2238959908032,0.641061424759933));
#10247=CARTESIAN_POINT('Ctrl Pts',(0.900002662567364,1.22064256379503,0.648296551655426));
#10248=CARTESIAN_POINT('Ctrl Pts',(0.900001146653719,1.21656554418039,0.655104870690721));
#10249=CARTESIAN_POINT('Ctrl Pts',(0.900000540233788,1.21172928299109,0.66132323772617));
#10250=CARTESIAN_POINT('Ctrl Pts',(0.900000424918953,1.21080963534652,0.66250570210793));
#10251=CARTESIAN_POINT('Ctrl Pts',(0.900000351402035,1.20986240082127,0.663666762843393));
#10252=CARTESIAN_POINT('Ctrl Pts',(0.900000346234225,1.20888784277449,0.664805176146358));
#10253=CARTESIAN_POINT('Ctrl Pts',(0.900000336405833,1.20703438079614,0.666970266034709));
#10254=CARTESIAN_POINT('Ctrl Pts',(0.900000571869483,1.20508211779724,0.669053482241208));
#10255=CARTESIAN_POINT('Ctrl Pts',(0.900000903580486,1.20303784749416,0.671051418948595));
#10256=CARTESIAN_POINT('Ctrl Pts',(0.900001825932764,1.19735357006848,0.676606861644505));
#10257=CARTESIAN_POINT('Ctrl Pts',(0.900003332967427,1.19102482074992,0.681443262092019));
#10258=CARTESIAN_POINT('Ctrl Pts',(0.900003895332687,1.18421635668109,0.685507797106414));
#10259=CARTESIAN_POINT('Ctrl Pts',(0.900004254598985,1.17986677848026,0.688104419886002));
#10260=CARTESIAN_POINT('Ctrl Pts',(0.9000042929279,1.17532044218795,0.69038534615497));
#10261=CARTESIAN_POINT('Ctrl Pts',(0.900003997675654,1.17061445353731,0.692327416690341));
#10262=CARTESIAN_POINT('Ctrl Pts',(0.900003537640084,1.16328200409216,0.695353376818313));
#10263=CARTESIAN_POINT('Ctrl Pts',(0.900002259964378,1.15564663185935,0.697524398440697));
#10264=CARTESIAN_POINT('Ctrl Pts',(0.900001215101098,1.14785635641255,0.698771715080855));
#10265=CARTESIAN_POINT('Ctrl Pts',(0.900000537649455,1.14280542295857,0.699580430175527));
#10266=CARTESIAN_POINT('Ctrl Pts',(0.899999997568109,1.13768876957788,0.699999998835552));
#10267=CARTESIAN_POINT('Ctrl Pts',(0.899999999937205,1.13254484130906,0.7));
#10268=CARTESIAN_POINT('Ctrl Pts',(0.9,1.266106713614,0.));
#10269=CARTESIAN_POINT('Ctrl Pts',(0.9,1.26053025554556,0.100869097599589));
#10270=CARTESIAN_POINT('Ctrl Pts',(0.9,1.25495230648558,0.201739398169819));
#10271=CARTESIAN_POINT('Ctrl Pts',(0.9,1.24378819189631,0.403576374532447));
#10272=CARTESIAN_POINT('Ctrl Pts',(0.9,1.23820188085298,0.504545629805417));
#10273=CARTESIAN_POINT('Ctrl Pts',(0.9,1.23261418131727,0.605513513251856));
#10274=CARTESIAN_POINT('Ctrl Pts',(0.900000000000002,-1.266106713614,-8.15320033709099E-17));
#10275=CARTESIAN_POINT('Ctrl Pts',(0.908871090277923,-1.25552568177643,
0.201930159665972));
#10276=CARTESIAN_POINT('Ctrl Pts',(0.917742329685194,-1.24494466498547,
0.403860313587921));
#10277=CARTESIAN_POINT('Ctrl Pts',(0.926613720860141,-1.23436366359623,
0.605790461668883));
#10278=CARTESIAN_POINT('Ctrl Pts',(0.697441255022372,-1.25280938151844,
-5.71013218131409E-5));
#10279=CARTESIAN_POINT('Ctrl Pts',(0.706712389899261,-1.24222855501813,
0.201872952723963));
#10280=CARTESIAN_POINT('Ctrl Pts',(0.71598368260269,-1.23164774534186,0.403803000441224));
#10281=CARTESIAN_POINT('Ctrl Pts',(0.725255135891715,-1.22106695288555,
0.605733041729342));
#10282=CARTESIAN_POINT('Ctrl Pts',(0.494899146035781,-1.23832021354117,
-0.000119230777047918));
#10283=CARTESIAN_POINT('Ctrl Pts',(0.504570354086872,-1.2277396148863,0.201810708652083));
#10284=CARTESIAN_POINT('Ctrl Pts',(0.514241728780064,-1.21715903502506,
0.403740641123913));
#10285=CARTESIAN_POINT('Ctrl Pts',(0.523913273026478,-1.20657847439907,
0.605670566527588));
#10286=CARTESIAN_POINT('Ctrl Pts',(0.292373353339556,-1.22258574808743,
-0.000186633859775947));
#10287=CARTESIAN_POINT('Ctrl Pts',(0.302444661323169,-1.21200540195431,
0.201743181663441));
#10288=CARTESIAN_POINT('Ctrl Pts',(0.312516144861689,-1.20142507679253,
0.403672989556125));
#10289=CARTESIAN_POINT('Ctrl Pts',(0.322587807049886,-1.190844773096,0.605602789690272));
#10290=CARTESIAN_POINT('',(0.32407846024449,-1.19096124572524,0.605603291426262));
#10291=CARTESIAN_POINT('Ctrl Pts',(0.292382661757373,-1.22257596919059,
-1.26634813746307E-16));
#10292=CARTESIAN_POINT('Ctrl Pts',(0.302948004341657,-1.21203750712027,
0.201867748891544));
#10293=CARTESIAN_POINT('Ctrl Pts',(0.313513270922098,-1.20149926476964,
0.403735512620674));
#10294=CARTESIAN_POINT('Ctrl Pts',(0.324078460244491,-1.19096124572524,
0.605603291426262));
#10295=CARTESIAN_POINT('Ctrl Pts',(0.324078460244487,-1.19096124572524,
0.605603291426262));
#10296=CARTESIAN_POINT('Ctrl Pts',(0.515976798438381,-1.20595780001216,
0.605571001180369));
#10297=CARTESIAN_POINT('Ctrl Pts',(0.707956283694857,-1.21982772882273,
0.605541108414459));
#10298=CARTESIAN_POINT('Ctrl Pts',(0.900000000000001,-1.23261418131727,
0.605513513251856));
#10299=CARTESIAN_POINT('Ctrl Pts',(0.906632491847682,-1.13298681949577,
0.7));
#10300=CARTESIAN_POINT('Ctrl Pts',(0.714963137593258,-1.12022681655782,
0.7));
#10301=CARTESIAN_POINT('Ctrl Pts',(0.52336552158394,-1.10638609587519,0.7));
#10302=CARTESIAN_POINT('Ctrl Pts',(0.331856371369197,-1.09142177001972,
0.7));
#10303=CARTESIAN_POINT('Ctrl Pts',(0.904714827274509,-1.16179226195561,
0.7));
#10304=CARTESIAN_POINT('Ctrl Pts',(0.712937153454425,-1.14901967286075,
0.69999980360337));
#10305=CARTESIAN_POINT('Ctrl Pts',(0.521230340369869,-1.13516557394852,
0.700000229443053));
#10306=CARTESIAN_POINT('Ctrl Pts',(0.329608751265076,-1.12018616744754,
0.7));
#10307=CARTESIAN_POINT('Ctrl Pts',(0.901389714107723,-1.21173913866089,
0.676722045797292));
#10308=CARTESIAN_POINT('Ctrl Pts',(0.709425477581998,-1.19894546296063,
0.676731074746188));
#10309=CARTESIAN_POINT('Ctrl Pts',(0.517526696841433,-1.18506766126723,
0.67674067107047));
#10310=CARTESIAN_POINT('Ctrl Pts',(0.325711429829026,-1.17006296935233,
0.676751229163451));
#10311=CARTESIAN_POINT('Ctrl Pts',(0.900079298017777,-1.23142303740181,
0.627132481749528));
#10312=CARTESIAN_POINT('Ctrl Pts',(0.708040181852795,-1.21863106773591,
0.627155851652593));
#10313=CARTESIAN_POINT('Ctrl Pts',(0.516066269599777,-1.20475540724405,
0.627181012790208));
#10314=CARTESIAN_POINT('Ctrl Pts',(0.324172915772929,-1.18975243096407,
0.627208352638976));
#10315=CARTESIAN_POINT('Ctrl Pts',(0.900000000000001,-1.23261418131727,
0.605513513251856));
#10316=CARTESIAN_POINT('Ctrl Pts',(0.707956283694857,-1.21982772882273,
0.605541108414459));
#10317=CARTESIAN_POINT('Ctrl Pts',(0.515976798438381,-1.20595780001216,
0.605571001180369));
#10318=CARTESIAN_POINT('Ctrl Pts',(0.324078460244487,-1.19096124572524,
0.605603291426262));
#10319=CARTESIAN_POINT('',(0.3318563713692,-1.09142177001972,0.7));
#10320=CARTESIAN_POINT('Origin',(0.3318563713692,-1.09142177001972,0.6));
#10321=CARTESIAN_POINT('Ctrl Pts',(0.899999999937167,-1.13254484130906,
0.7));
#10322=CARTESIAN_POINT('Ctrl Pts',(0.710543123935439,-1.11990737114256,
0.7));
#10323=CARTESIAN_POINT('Ctrl Pts',(0.521156529292483,-1.10621348751457,
0.7));
#10324=CARTESIAN_POINT('Ctrl Pts',(0.331856371369197,-1.09142177001972,
0.7));
#10325=CARTESIAN_POINT('Origin',(5.4,-8.11656130105013E-18,0.7));
#10326=CARTESIAN_POINT('',(0.3318563713692,1.09142177001972,0.7));
#10327=CARTESIAN_POINT('',(0.3318563713692,-0.7,0.7));
#10328=CARTESIAN_POINT('Ctrl Pts',(0.3318563713692,1.09142177001972,0.7));
#10329=CARTESIAN_POINT('Ctrl Pts',(0.521156529292483,1.10621348751457,0.7));
#10330=CARTESIAN_POINT('Ctrl Pts',(0.710543123935438,1.11990737114256,0.7));
#10331=CARTESIAN_POINT('Ctrl Pts',(0.899999999937165,1.13254484130906,0.7));
#10332=CARTESIAN_POINT('Ctrl Pts',(0.292373353339556,1.22258574808743,-0.000186633859776018));
#10333=CARTESIAN_POINT('Ctrl Pts',(0.30244466132317,1.21200540195431,0.20174318166344));
#10334=CARTESIAN_POINT('Ctrl Pts',(0.31251614486169,1.20142507679253,0.403672989556124));
#10335=CARTESIAN_POINT('Ctrl Pts',(0.322587807049886,1.190844773096,0.605602789690271));
#10336=CARTESIAN_POINT('Ctrl Pts',(0.494899146035781,1.23832021354117,-0.000119230777047989));
#10337=CARTESIAN_POINT('Ctrl Pts',(0.504570354086872,1.2277396148863,0.201810708652083));
#10338=CARTESIAN_POINT('Ctrl Pts',(0.514241728780064,1.21715903502506,0.403740641123914));
#10339=CARTESIAN_POINT('Ctrl Pts',(0.523913273026478,1.20657847439907,0.605670566527587));
#10340=CARTESIAN_POINT('Ctrl Pts',(0.697441255022371,1.25280938151844,-5.71013218130602E-5));
#10341=CARTESIAN_POINT('Ctrl Pts',(0.70671238989926,1.24222855501813,0.201872952723963));
#10342=CARTESIAN_POINT('Ctrl Pts',(0.715983682602689,1.23164774534186,0.403803000441224));
#10343=CARTESIAN_POINT('Ctrl Pts',(0.725255135891714,1.22106695288555,0.605733041729342));
#10344=CARTESIAN_POINT('Ctrl Pts',(0.9,1.266106713614,1.73472347597681E-18));
#10345=CARTESIAN_POINT('Ctrl Pts',(0.908871090277921,1.25552568177643,0.201930159665973));
#10346=CARTESIAN_POINT('Ctrl Pts',(0.917742329685192,1.24494466498547,0.403860313587921));
#10347=CARTESIAN_POINT('Ctrl Pts',(0.92661372086014,1.23436366359623,0.605790461668883));
#10348=CARTESIAN_POINT('',(0.32407846024449,1.19096124572524,0.605603291426262));
#10349=CARTESIAN_POINT('Ctrl Pts',(0.9,1.23261418131727,0.605513513251856));
#10350=CARTESIAN_POINT('Ctrl Pts',(0.707956283694857,1.21982772882273,0.605541108414459));
#10351=CARTESIAN_POINT('Ctrl Pts',(0.515976798438382,1.20595780001216,0.60557100118037));
#10352=CARTESIAN_POINT('Ctrl Pts',(0.32407846024449,1.19096124572524,0.605603291426262));
#10353=CARTESIAN_POINT('Ctrl Pts',(0.324078460244491,1.19096124572524,0.605603291426262));
#10354=CARTESIAN_POINT('Ctrl Pts',(0.313513270922098,1.20149926476964,0.403735512620674));
#10355=CARTESIAN_POINT('Ctrl Pts',(0.302948004341658,1.21203750712026,0.201867748891544));
#10356=CARTESIAN_POINT('Ctrl Pts',(0.292382661757373,1.22257596919059,3.4477629085039E-17));
#10357=CARTESIAN_POINT('Ctrl Pts',(0.3318563713692,1.09142177001972,0.7));
#10358=CARTESIAN_POINT('Ctrl Pts',(0.523365521583941,1.10638609587519,0.7));
#10359=CARTESIAN_POINT('Ctrl Pts',(0.714963137593258,1.12022681655782,0.7));
#10360=CARTESIAN_POINT('Ctrl Pts',(0.906632491847681,1.13298681949577,0.7));
#10361=CARTESIAN_POINT('Ctrl Pts',(0.329608751265078,1.12018616744754,0.7));
#10362=CARTESIAN_POINT('Ctrl Pts',(0.52123034036987,1.13516557394852,0.700000229443053));
#10363=CARTESIAN_POINT('Ctrl Pts',(0.712937153454426,1.14901967286075,0.699999803603371));
#10364=CARTESIAN_POINT('Ctrl Pts',(0.904714827274509,1.16179226195561,0.700000000000001));
#10365=CARTESIAN_POINT('Ctrl Pts',(0.325711429829028,1.17006296935233,0.676751229163452));
#10366=CARTESIAN_POINT('Ctrl Pts',(0.517526696841433,1.18506766126723,0.67674067107047));
#10367=CARTESIAN_POINT('Ctrl Pts',(0.709425477581997,1.19894546296063,0.676731074746189));
#10368=CARTESIAN_POINT('Ctrl Pts',(0.901389714107722,1.21173913866089,0.676722045797292));
#10369=CARTESIAN_POINT('Ctrl Pts',(0.324172915772932,1.18975243096407,0.627208352638976));
#10370=CARTESIAN_POINT('Ctrl Pts',(0.516066269599778,1.20475540724405,0.627181012790208));
#10371=CARTESIAN_POINT('Ctrl Pts',(0.708040181852794,1.21863106773591,0.627155851652593));
#10372=CARTESIAN_POINT('Ctrl Pts',(0.900079298017776,1.23142303740181,0.627132481749528));
#10373=CARTESIAN_POINT('Ctrl Pts',(0.32407846024449,1.19096124572524,0.605603291426262));
#10374=CARTESIAN_POINT('Ctrl Pts',(0.515976798438382,1.20595780001216,0.60557100118037));
#10375=CARTESIAN_POINT('Ctrl Pts',(0.707956283694857,1.21982772882273,0.605541108414459));
#10376=CARTESIAN_POINT('Ctrl Pts',(0.9,1.23261418131727,0.605513513251856));
#10377=CARTESIAN_POINT('Origin',(0.331856371369202,1.09142177001972,0.6));
#10378=CARTESIAN_POINT('Origin',(0.331856371369202,1.09142177001972,0.6));
#10379=CARTESIAN_POINT('Origin',(0.331856371369201,1.09142177001972,0.6));
#10380=CARTESIAN_POINT('Origin',(0.331856371369202,1.09142177001972,0.6));
#10381=CARTESIAN_POINT('Origin',(10.4681436286308,1.08420482079361,0.6));
#10382=CARTESIAN_POINT('Origin',(10.4681436276939,1.08420482084454,0.6));
#10383=CARTESIAN_POINT('',(10.5680065821063,1.08420482079361,0.605233595624295));
#10384=CARTESIAN_POINT('Origin',(10.4681436286308,1.08420482079361,0.6));
#10385=CARTESIAN_POINT('Origin',(10.4681436286308,1.08420482079361,0.6));
#10386=CARTESIAN_POINT('Origin',(0.3318563713692,-1.09142177001972,0.6));
#10387=CARTESIAN_POINT('Origin',(0.331856371369201,-1.09142177001972,0.6));
#10388=CARTESIAN_POINT('Origin',(0.3318563713692,-1.09142177001972,0.6));
#10389=CARTESIAN_POINT('Origin',(0.3318563713692,-0.7,0.6));
#10390=CARTESIAN_POINT('Ctrl Pts',(0.2922895713475,-1.22266882276207,-0.00177864096060679));
#10391=CARTESIAN_POINT('Ctrl Pts',(0.302885944515497,-1.21209940820877,
0.200681988163859));
#10392=CARTESIAN_POINT('Ctrl Pts',(0.313482241236256,-1.20153021465708,
0.403142632212487));
#10393=CARTESIAN_POINT('Ctrl Pts',(0.324078460244491,-1.19096124572524,
0.605603291426262));
#10394=CARTESIAN_POINT('Ctrl Pts',(0.264022491930188,-1.22039553779506,
-0.000415890128406236));
#10395=CARTESIAN_POINT('Ctrl Pts',(0.274621881512248,-1.20982222712748,
0.202044379074236));
#10396=CARTESIAN_POINT('Ctrl Pts',(0.285221154833576,-1.19924944554801,
0.404504681968985));
#10397=CARTESIAN_POINT('Ctrl Pts',(0.29582042516239,-1.18867654001483,0.606964977361795));
#10398=CARTESIAN_POINT('Ctrl Pts',(0.216712469170969,-1.1940874043406,0.000690255297866666));
#10399=CARTESIAN_POINT('Ctrl Pts',(0.227319688237882,-1.18351239299796,
0.203150045648192));
#10400=CARTESIAN_POINT('Ctrl Pts',(0.237926932441998,-1.17293746916702,
0.405609838636422));
#10401=CARTESIAN_POINT('Ctrl Pts',(0.248534117816369,-1.1623628476683,0.608069650238703));
#10402=CARTESIAN_POINT('Ctrl Pts',(0.200219987929043,-1.14439035743082,
-0.00103956457010847));
#10403=CARTESIAN_POINT('Ctrl Pts',(0.210830491339948,-1.13382006821851,
0.201420337884579));
#10404=CARTESIAN_POINT('Ctrl Pts',(0.221440906577676,-1.12324995278282,
0.403880253819325));
#10405=CARTESIAN_POINT('Ctrl Pts',(0.232051411471599,-1.11268010558856,
0.606340179010355));
#10406=CARTESIAN_POINT('Ctrl Pts',(0.200161975173303,-1.12312592850316,
-0.00214651389202307));
#10407=CARTESIAN_POINT('Ctrl Pts',(0.210772455448684,-1.11255764422181,
0.200313510564959));
#10408=CARTESIAN_POINT('Ctrl Pts',(0.221382936352032,-1.1019895901204,0.402773547004277));
#10409=CARTESIAN_POINT('Ctrl Pts',(0.231993417893744,-1.09142177001972,
0.605233595624295));
#10410=CARTESIAN_POINT('Origin',(10.4681436286308,-1.08420482109828,0.6));
#10411=CARTESIAN_POINT('',(10.5680065821063,-1.08420482079361,0.605233595624295));
#10412=CARTESIAN_POINT('Origin',(10.4681436286308,-1.08420482099672,0.600000000000001));
#10413=CARTESIAN_POINT('Origin',(10.4681436286308,-1.08420482109828,0.6));
#10414=CARTESIAN_POINT('Origin',(10.4681436286308,0.7,0.6));
#10415=CARTESIAN_POINT('',(10.5680065821063,0.7,0.605233595624295));
#10416=CARTESIAN_POINT('Ctrl Pts',(10.599839982685,-1.11594741464673,-0.00218387205330164));
#10417=CARTESIAN_POINT('Ctrl Pts',(10.5892288496247,-1.10536637943871,0.200288608282177));
#10418=CARTESIAN_POINT('Ctrl Pts',(10.5786177161011,-1.0947855138519,0.402761097457634));
#10419=CARTESIAN_POINT('Ctrl Pts',(10.5680065821063,-1.08420482079362,0.605233595624295));
#10420=CARTESIAN_POINT('Ctrl Pts',(10.5997613205547,-1.14474784499259,-0.000682909193257743));
#10421=CARTESIAN_POINT('Ctrl Pts',(10.5891501209488,-1.13416481604349,0.201789447273867));
#10422=CARTESIAN_POINT('Ctrl Pts',(10.5785391399155,-1.12358205581644,0.404261829287571));
#10423=CARTESIAN_POINT('Ctrl Pts',(10.5679279386544,-1.11299934606825,0.606734202078189));
#10424=CARTESIAN_POINT('Ctrl Pts',(10.5764119435127,-1.19466846760808,0.000702210001053139));
#10425=CARTESIAN_POINT('Ctrl Pts',(10.5658041809617,-1.18408222297768,0.203174550667819));
#10426=CARTESIAN_POINT('Ctrl Pts',(10.5551963844732,-1.17349608774572,0.405646894856767));
#10427=CARTESIAN_POINT('Ctrl Pts',(10.544588659013,-1.16291012508165,0.608119251464957));
#10428=CARTESIAN_POINT('Ctrl Pts',(10.5269342003857,-1.21442651155969,-0.000858270497959616));
#10429=CARTESIAN_POINT('Ctrl Pts',(10.5163317654776,-1.20384274018949,0.201614467507756));
#10430=CARTESIAN_POINT('Ctrl Pts',(10.5057293269973,-1.1932591813998,0.404087216090532));
#10431=CARTESIAN_POINT('Ctrl Pts',(10.4951269905998,-1.18267571840064,0.606559974437339));
#10432=CARTESIAN_POINT('Ctrl Pts',(10.5053655128635,-1.21565094114741,-0.0019246498908503));
#10433=CARTESIAN_POINT('Ctrl Pts',(10.4947646468921,-1.20506932615592,0.200548282383137));
#10434=CARTESIAN_POINT('Ctrl Pts',(10.4841638390504,-1.19448787589602,0.403021225840181));
#10435=CARTESIAN_POINT('Ctrl Pts',(10.4735630903435,-1.18390659316268,0.605494180667945));
#10436=CARTESIAN_POINT('Ctrl Pts',(10.5997255308004,-1.11583328740478,1.02782365951626E-16));
#10437=CARTESIAN_POINT('Ctrl Pts',(10.589152548365,-1.10529029582828,0.201744523047832));
#10438=CARTESIAN_POINT('Ctrl Pts',(10.5785795654695,-1.09474747266587,0.40348905487273));
#10439=CARTESIAN_POINT('Ctrl Pts',(10.5680065821063,-1.08420482079362,0.605233595624295));
#10440=CARTESIAN_POINT('Ctrl Pts',(10.5053638082297,1.21564923960921,-0.0018920919656423));
#10441=CARTESIAN_POINT('Ctrl Pts',(10.4947635104759,1.20506819181477,0.200569987667808));
#10442=CARTESIAN_POINT('Ctrl Pts',(10.4841632708454,1.19448730873444,0.403032078483127));
#10443=CARTESIAN_POINT('Ctrl Pts',(10.4735630903435,1.18390659316268,0.605494180667945));
#10444=CARTESIAN_POINT('Ctrl Pts',(10.5341220579192,1.21401666636749,-0.000470252816738081));
#10445=CARTESIAN_POINT('Ctrl Pts',(10.5235196325477,1.20343268662274,0.201991562854702));
#10446=CARTESIAN_POINT('Ctrl Pts',(10.5129172908767,1.19284910679518,0.404453403808947));
#10447=CARTESIAN_POINT('Ctrl Pts',(10.5023149573519,1.18226542681329,0.606915239027137));
#10448=CARTESIAN_POINT('Ctrl Pts',(10.5827170203615,1.18801090922716,0.000717463067903341));
#10449=CARTESIAN_POINT('Ctrl Pts',(10.5721088691741,1.17742555398174,0.203178921531494));
#10450=CARTESIAN_POINT('Ctrl Pts',(10.5615007184277,1.16684027916303,0.405640383775807));
#10451=CARTESIAN_POINT('Ctrl Pts',(10.5508925935528,1.15625520969485,0.60810185787831));
#10452=CARTESIAN_POINT('Ctrl Pts',(10.5997792798033,1.13754603572512,-0.00102559206997387));
#10453=CARTESIAN_POINT('Ctrl Pts',(10.5891686973038,1.12696411138589,0.201435946515793));
#10454=CARTESIAN_POINT('Ctrl Pts',(10.5785581831385,1.11638231376635,0.40389749513889));
#10455=CARTESIAN_POINT('Ctrl Pts',(10.5679475995174,1.10580071474959,0.606359050464716));
#10456=CARTESIAN_POINT('Ctrl Pts',(10.5998382764002,1.11594571320176,-0.00215131420076595));
#10457=CARTESIAN_POINT('Ctrl Pts',(10.5892277121014,1.10536524516024,0.200310313518148));
#10458=CARTESIAN_POINT('Ctrl Pts',(10.5786171473394,1.09478494672192,0.402771950076102));
#10459=CARTESIAN_POINT('Ctrl Pts',(10.5680065821063,1.08420482079361,0.605233595624295));
#10460=CARTESIAN_POINT('Ctrl Pts',(10.5680065821063,1.08420482079361,0.605233595624295));
#10461=CARTESIAN_POINT('Ctrl Pts',(10.5785795654695,1.09474747266587,0.40348905487273));
#10462=CARTESIAN_POINT('Ctrl Pts',(10.589152548365,1.10529029582828,0.201744523047831));
#10463=CARTESIAN_POINT('Ctrl Pts',(10.5997255308004,1.11583328740478,1.07661275727811E-16));
#10464=CARTESIAN_POINT('Ctrl Pts',(10.1947388861048,1.09885088260187,0.7));
#10465=CARTESIAN_POINT('Ctrl Pts',(10.285877616441,1.09404209584202,0.7));
#10466=CARTESIAN_POINT('Ctrl Pts',(10.3770124662346,1.0891584122264,0.7));
#10467=CARTESIAN_POINT('Ctrl Pts',(10.4681436286308,1.08420482079361,0.7));
#10468=CARTESIAN_POINT('Ctrl Pts',(10.196260416419,1.12768774893097,0.700000000000001));
#10469=CARTESIAN_POINT('Ctrl Pts',(10.2874149314686,1.12287675076168,0.699999949550842));
#10470=CARTESIAN_POINT('Ctrl Pts',(10.3785648662465,1.11799094453753,0.700000051218742));
#10471=CARTESIAN_POINT('Ctrl Pts',(10.4697107510168,1.11303515260326,0.7));
#10472=CARTESIAN_POINT('Ctrl Pts',(10.1988975981852,1.17766904563614,0.67669140632491));
#10473=CARTESIAN_POINT('Ctrl Pts',(10.2900793016129,1.17285439035486,0.676693724638983));
#10474=CARTESIAN_POINT('Ctrl Pts',(10.3812557252598,1.16796482352885,0.676696026813929));
#10475=CARTESIAN_POINT('Ctrl Pts',(10.4724269697127,1.16300539549315,0.676698381019544));
#10476=CARTESIAN_POINT('Ctrl Pts',(10.1999375452555,1.19737868557977,0.627098033786781));
#10477=CARTESIAN_POINT('Ctrl Pts',(10.2911301919381,1.19256517083271,0.627104033151799));
#10478=CARTESIAN_POINT('Ctrl Pts',(10.382317043787,1.18767684023183,0.627110048826767));
#10479=CARTESIAN_POINT('Ctrl Pts',(10.4734985149421,1.18271860027509,0.627116141711795));
#10480=CARTESIAN_POINT('Ctrl Pts',(10.1999999975038,1.19856231440453,0.605472757505366));
#10481=CARTESIAN_POINT('Ctrl Pts',(10.2911933328565,1.19375025772558,0.605479840815741));
#10482=CARTESIAN_POINT('Ctrl Pts',(10.3823809652617,1.18886335120032,0.605486986548286));
#10483=CARTESIAN_POINT('Ctrl Pts',(10.4735630903435,1.18390659316268,0.605494180667944));
#10484=CARTESIAN_POINT('Ctrl Pts',(0.200159601751749,1.12312829248604,-0.00219180147311912));
#10485=CARTESIAN_POINT('Ctrl Pts',(0.210770873167554,1.11255922017607,0.200283318842441));
#10486=CARTESIAN_POINT('Ctrl Pts',(0.221382145211419,1.10199037808008,0.402758451142111));
#10487=CARTESIAN_POINT('Ctrl Pts',(0.231993417893744,1.09142177001972,0.605233595624295));
#10488=CARTESIAN_POINT('Ctrl Pts',(0.200236952094631,1.15148086499205,-0.000715869007730825));
#10489=CARTESIAN_POINT('Ctrl Pts',(0.210848310847714,1.14090905181173,0.201759082033021));
#10490=CARTESIAN_POINT('Ctrl Pts',(0.221459381762758,1.13033759660317,0.404234066901971));
#10491=CARTESIAN_POINT('Ctrl Pts',(0.232070742664217,1.11976621744484,0.606709040139042));
#10492=CARTESIAN_POINT('Ctrl Pts',(0.222806696702742,1.20067708175657,0.000669311976984441));
#10493=CARTESIAN_POINT('Ctrl Pts',(0.233413416075889,1.19010082554658,0.203144236955742));
#10494=CARTESIAN_POINT('Ctrl Pts',(0.244020198555212,1.17952469009474,0.405619164345205));
#10495=CARTESIAN_POINT('Ctrl Pts',(0.254626870458834,1.16894881850735,0.608094110943904));
#10496=CARTESIAN_POINT('Ctrl Pts',(0.271086891015657,1.22096622390789,-0.000801865493577694));
#10497=CARTESIAN_POINT('Ctrl Pts',(0.281686280594249,1.21039315447922,0.201673594461172));
#10498=CARTESIAN_POINT('Ctrl Pts',(0.292285672737775,1.1998203699977,0.404149068703718));
#10499=CARTESIAN_POINT('Ctrl Pts',(0.302884933932915,1.18924771644243,0.606624555877912));
#10500=CARTESIAN_POINT('Ctrl Pts',(0.292287201081515,1.22267118699778,-0.00182392867695869));
#10501=CARTESIAN_POINT('Ctrl Pts',(0.302884364349574,1.21210098433295,0.200651796350731));
#10502=CARTESIAN_POINT('Ctrl Pts',(0.313481451159089,1.20153100270242,0.403127536304793));
#10503=CARTESIAN_POINT('Ctrl Pts',(0.324078460244491,1.19096124572524,0.605603291426262));
#10504=CARTESIAN_POINT('Origin',(10.6002740930491,1.4,-0.0104671912485891));
#10505=CARTESIAN_POINT('Origin',(0.331856371369202,1.09142177001972,0.6));
#10506=CARTESIAN_POINT('',(0.3318563713692,1.09142177001972,0.9));
#10507=CARTESIAN_POINT('',(0.0322675109428288,1.09142177001972,0.615700786872883));
#10508=CARTESIAN_POINT('Origin',(0.3318563713692,1.09142177001972,0.6));
#10509=CARTESIAN_POINT('',(0.308522637995069,1.39004019713626,0.616809874278785));
#10510=CARTESIAN_POINT('Origin',(0.331856371369202,1.09142177001972,0.6));
#10511=CARTESIAN_POINT('Origin',(0.331856371369201,1.09142177001972,0.6));
#10512=CARTESIAN_POINT('Origin',(10.4681436286308,1.08420482079361,0.6));
#10513=CARTESIAN_POINT('',(10.4681436286308,1.08420482109828,0.9));
#10514=CARTESIAN_POINT('',(10.4844020137689,1.3833101379008,0.616482542003833));
#10515=CARTESIAN_POINT('Origin',(10.4681436258201,1.08420482094639,0.6));
#10516=CARTESIAN_POINT('',(10.7677324890572,1.08420482079361,0.615700786872884));
#10517=CARTESIAN_POINT('Origin',(10.4681436286308,1.08420482079361,0.6));
#10518=CARTESIAN_POINT('Origin',(10.4681436286308,1.08420482079362,0.6));
#10519=CARTESIAN_POINT('Origin',(0.3318563713692,-1.09142177001972,0.6));
#10520=CARTESIAN_POINT('',(0.3318563713692,-1.09142177001972,0.9));
#10521=CARTESIAN_POINT('',(0.308522637995069,-1.39004019713626,0.616809874278785));
#10522=CARTESIAN_POINT('Origin',(0.3318563713692,-1.09142177001972,0.6));
#10523=CARTESIAN_POINT('',(0.0322675109428289,-1.09142177001972,0.615700786872884));
#10524=CARTESIAN_POINT('Origin',(0.3318563713692,-1.09142177001972,0.6));
#10525=CARTESIAN_POINT('Origin',(0.331856371369201,-1.09142177001972,0.6));
#10526=CARTESIAN_POINT('Origin',(0.3318563713692,-0.7,0.6));
#10527=CARTESIAN_POINT('',(0.0322675109428288,-0.7,0.615700786872883));
#10528=CARTESIAN_POINT('',(0.3318563713692,-0.7,0.9));
#10529=CARTESIAN_POINT('Ctrl Pts',(0.276048389810261,-1.42252533450788,
-0.00533608639730399));
#10530=CARTESIAN_POINT('Ctrl Pts',(0.28687338241706,-1.4116967417008,0.202045878554724));
#10531=CARTESIAN_POINT('Ctrl Pts',(0.297698133178874,-1.40086836142621,
0.409427865329919));
#10532=CARTESIAN_POINT('Ctrl Pts',(0.308522637995069,-1.39004019713626,
0.616809874278785));
#10533=CARTESIAN_POINT('Ctrl Pts',(0.191246496057484,-1.41570630783033,
-0.00124775669238285));
#10534=CARTESIAN_POINT('Ctrl Pts',(0.202080757839133,-1.40486573978029,
0.206133102090467));
#10535=CARTESIAN_POINT('Ctrl Pts',(0.212914648880055,-1.39402634701096,
0.413514041581016));
#10536=CARTESIAN_POINT('Ctrl Pts',(0.223748532748767,-1.38318608000504,
0.620894932085382));
#10537=CARTESIAN_POINT('Ctrl Pts',(0.0492682973509243,-1.33685850703924,
0.00207719607616587));
#10538=CARTESIAN_POINT('Ctrl Pts',(0.0601266125734448,-1.32601270457081,
0.209456583216085));
#10539=CARTESIAN_POINT('Ctrl Pts',(0.0709850253737815,-1.3151666447344,
0.416835949794532));
#10540=CARTESIAN_POINT('Ctrl Pts',(0.0818432319483421,-1.30432109509162,
0.624215353109623));
#10541=CARTESIAN_POINT('Ctrl Pts',(-0.000163444061205068,-1.18769013309795,
-0.00311869847265479));
#10542=CARTESIAN_POINT('Ctrl Pts',(0.0107049555364969,-1.17685886333949,
0.204261034729081));
#10543=CARTESIAN_POINT('Ctrl Pts',(0.0215730900970294,-1.16602762920277,
0.411640782964944));
#10544=CARTESIAN_POINT('Ctrl Pts',(0.0324414916763936,-1.15519677672624,
0.619020537031064));
#10545=CARTESIAN_POINT('Ctrl Pts',(-0.00033748371827097,-1.12389640457412,
-0.0064395729582146));
#10546=CARTESIAN_POINT('Ctrl Pts',(0.0105308471731094,-1.11307128361434,
0.200940534347673));
#10547=CARTESIAN_POINT('Ctrl Pts',(0.0213991787230862,-1.10224640406117,
0.408320654220332));
#10548=CARTESIAN_POINT('Ctrl Pts',(0.0322675109428289,-1.09142177001972,
0.615700786872884));
#10549=CARTESIAN_POINT('Ctrl Pts',(0.27632692456468,-1.42224670711126,5.13911829758129E-17));
#10550=CARTESIAN_POINT('Ctrl Pts',(0.287059068122268,-1.41151099373342,
0.20560326985903));
#10551=CARTESIAN_POINT('Ctrl Pts',(0.297790973931072,-1.40077548928706,
0.411206561171438));
#10552=CARTESIAN_POINT('Ctrl Pts',(0.308522637995069,-1.39004019713626,
0.616809874278785));
#10553=CARTESIAN_POINT('Ctrl Pts',(0.0322675109428289,-1.09142177001972,
0.615700786872884));
#10554=CARTESIAN_POINT('Ctrl Pts',(0.0215116733095221,-1.10213436178043,
0.410467178800746));
#10555=CARTESIAN_POINT('Ctrl Pts',(0.0107558363321879,-1.11284719399673,
0.205233583245308));
#10556=CARTESIAN_POINT('Ctrl Pts',(1.76901136968166E-16,-1.12356026268968,
-7.45931094670027E-17));
#10557=CARTESIAN_POINT('Origin',(10.4681436286308,-1.08420482109828,0.6));
#10558=CARTESIAN_POINT('',(10.7677324890572,-1.08420482079361,0.615700786872884));
#10559=CARTESIAN_POINT('',(10.4844020137689,-1.3833101379008,0.616482542003833));
#10560=CARTESIAN_POINT('Origin',(10.4681436286308,-1.08420482079361,0.600000000000001));
#10561=CARTESIAN_POINT('',(10.4681436258201,-1.08420482094639,0.9));
#10562=CARTESIAN_POINT('Origin',(10.4681436286308,-1.08420482109828,0.6));
#10563=CARTESIAN_POINT('Origin',(10.4681436286308,-1.08420482079361,0.6));
#10564=CARTESIAN_POINT('Origin',(10.4681436286308,0.7,0.6));
#10565=CARTESIAN_POINT('',(10.7677324890572,0.7,0.615700786872884));
#10566=CARTESIAN_POINT('',(10.4681436286308,0.7,0.9));
#10567=CARTESIAN_POINT('Ctrl Pts',(10.4681436286308,-1.08420482079361,0.9));
#10568=CARTESIAN_POINT('Ctrl Pts',(9.02115959826777,-1.16285813221549,0.9));
#10569=CARTESIAN_POINT('Ctrl Pts',(5.64262097844114,-1.30550334054488,0.9));
#10570=CARTESIAN_POINT('Ctrl Pts',(2.25816172369615,-1.24194126716656,0.9));
#10571=CARTESIAN_POINT('Ctrl Pts',(0.331856371369198,-1.09142177001972,
0.9));
#10572=CARTESIAN_POINT('Ctrl Pts',(10.4728449957889,-1.17069581622255,0.9));
#10573=CARTESIAN_POINT('Ctrl Pts',(9.02515960257209,-1.24945398332951,0.900002463983243));
#10574=CARTESIAN_POINT('Ctrl Pts',(5.64406008560805,-1.39235654229312,0.899995181674544));
#10575=CARTESIAN_POINT('Ctrl Pts',(2.25481214769604,-1.3286896492945,0.900006992415263));
#10576=CARTESIAN_POINT('Ctrl Pts',(0.325113511056834,-1.17771496230318,
0.9));
#10577=CARTESIAN_POINT('Ctrl Pts',(10.4809942371438,-1.32061731204901,0.830050158657121));
#10578=CARTESIAN_POINT('Ctrl Pts',(9.03210079995546,-1.3995487214628,0.829938185878055));
#10579=CARTESIAN_POINT('Ctrl Pts',(5.64656962219688,-1.54290142969263,0.82970437227026));
#10580=CARTESIAN_POINT('Ctrl Pts',(2.24896854757963,-1.47903552984056,0.829838703712927));
#10581=CARTESIAN_POINT('Ctrl Pts',(0.313425270489114,-1.32729771265557,
0.830156825336737));
#10582=CARTESIAN_POINT('Ctrl Pts',(10.4842082875648,-1.37974615923803,0.681348425135383));
#10583=CARTESIAN_POINT('Ctrl Pts',(9.03482793853036,-1.45862084618981,0.681058092399338));
#10584=CARTESIAN_POINT('Ctrl Pts',(5.64753778607331,-1.60187726023264,0.68045297450285));
#10585=CARTESIAN_POINT('Ctrl Pts',(2.24670449952385,-1.53809938127555,0.680799765935021));
#10586=CARTESIAN_POINT('Ctrl Pts',(0.308806004580392,-1.38641375285276,
0.681625057916928));
#10587=CARTESIAN_POINT('Ctrl Pts',(10.4844020137689,-1.3833101379008,0.616482542003833));
#10588=CARTESIAN_POINT('Ctrl Pts',(9.03499042108131,-1.46211428773623,0.616139856494792));
#10589=CARTESIAN_POINT('Ctrl Pts',(5.64759185703765,-1.60522711936681,0.615422163720642));
#10590=CARTESIAN_POINT('Ctrl Pts',(2.24657199659733,-1.54153220865049,0.615835494619844));
#10591=CARTESIAN_POINT('Ctrl Pts',(0.308522637995066,-1.39004019713626,
0.616809874278785));
#10592=CARTESIAN_POINT('Ctrl Pts',(0.308522637995066,-1.39004019713626,
0.616809874278785));
#10593=CARTESIAN_POINT('Ctrl Pts',(2.24657199659733,-1.54153220865049,0.615835494619844));
#10594=CARTESIAN_POINT('Ctrl Pts',(5.64759185703765,-1.60522711936681,0.615422163720642));
#10595=CARTESIAN_POINT('Ctrl Pts',(9.03499042108131,-1.46211428773623,0.616139856494792));
#10596=CARTESIAN_POINT('Ctrl Pts',(10.4844020137689,-1.3833101379008,0.616482542003833));
#10597=CARTESIAN_POINT('Ctrl Pts',(10.4681436258201,-1.08420482094639,0.900000000000001));
#10598=CARTESIAN_POINT('Ctrl Pts',(9.02115959639274,-1.16285813229465,0.9));
#10599=CARTESIAN_POINT('Ctrl Pts',(5.64262097750198,-1.30550334052724,0.9));
#10600=CARTESIAN_POINT('Ctrl Pts',(2.25816172369615,-1.24194126716656,0.9));
#10601=CARTESIAN_POINT('Ctrl Pts',(0.331856371369198,-1.09142177001972,
0.9));
#10602=CARTESIAN_POINT('Ctrl Pts',(10.8003433549902,-1.11672267507076,-0.00655160349952438));
#10603=CARTESIAN_POINT('Ctrl Pts',(10.7894730668347,-1.10588321133639,0.200865850630566));
#10604=CARTESIAN_POINT('Ctrl Pts',(10.7786027781932,-1.09504392553578,0.408283314033857));
#10605=CARTESIAN_POINT('Ctrl Pts',(10.7677324890572,-1.08420482079361,0.615700786872885));
#10606=CARTESIAN_POINT('Ctrl Pts',(10.8001073672393,-1.20312439623403,-0.00204868896805508));
#10607=CARTESIAN_POINT('Ctrl Pts',(10.7892368724076,-1.19227880391739,0.205368384315645));
#10608=CARTESIAN_POINT('Ctrl Pts',(10.7783670568079,-1.18143370221047,0.41278551899075));
#10609=CARTESIAN_POINT('Ctrl Pts',(10.7674965587017,-1.17058839661753,0.620202606234566));
#10610=CARTESIAN_POINT('Ctrl Pts',(10.7300137544668,-1.35289768637741,0.00210488808650419));
#10611=CARTESIAN_POINT('Ctrl Pts',(10.7191538066016,-1.34204221082848,0.209521911971666));
#10612=CARTESIAN_POINT('Ctrl Pts',(10.7082938463195,-1.33118673671862,0.416938933985702));
#10613=CARTESIAN_POINT('Ctrl Pts',(10.6974340169938,-1.32033143065575,0.624355970618915));
#10614=CARTESIAN_POINT('Ctrl Pts',(10.5816241002662,-1.4121605627967,-0.00257485550010117));
#10615=CARTESIAN_POINT('Ctrl Pts',(10.5707805459565,-1.4013126969686,0.204843391064434));
#10616=CARTESIAN_POINT('Ctrl Pts',(10.5599369567012,-1.39046512672587,0.412261650129749));
#10617=CARTESIAN_POINT('Ctrl Pts',(10.5490937145378,-1.37961751361469,0.619679923312015));
#10618=CARTESIAN_POINT('Ctrl Pts',(10.5169176890673,-1.41583338198674,-0.00577403633861717));
#10619=CARTESIAN_POINT('Ctrl Pts',(10.5060789456421,-1.40499213715574,0.201644806368331));
#10620=CARTESIAN_POINT('Ctrl Pts',(10.4952403861233,-1.39415105487295,0.40906366572247));
#10621=CARTESIAN_POINT('Ctrl Pts',(10.4844020137689,-1.3833101379008,0.616482542003833));
#10622=CARTESIAN_POINT('Ctrl Pts',(10.8,-1.11638029377732,-2.51534904016637E-17));
#10623=CARTESIAN_POINT('Ctrl Pts',(10.7892441634977,-1.10565496086826,0.205233586491178));
#10624=CARTESIAN_POINT('Ctrl Pts',(10.7784883265195,-1.09492980219801,0.410467182062988));
#10625=CARTESIAN_POINT('Ctrl Pts',(10.7677324890572,-1.08420482079361,0.615700786872885));
#10626=CARTESIAN_POINT('Ctrl Pts',(10.4844020137689,-1.3833101379008,0.616482542003833));
#10627=CARTESIAN_POINT('Ctrl Pts',(10.4951398148107,-1.39405045994841,0.410988344812119));
#10628=CARTESIAN_POINT('Ctrl Pts',(10.5058777995597,-1.40479094425298,0.205494164234945));
#10629=CARTESIAN_POINT('Ctrl Pts',(10.5166159648474,-1.4155315881283,-2.5652223401007E-16));
#10630=CARTESIAN_POINT('Ctrl Pts',(10.5169125872774,1.41582827901939,-0.0056764044152427));
#10631=CARTESIAN_POINT('Ctrl Pts',(10.5060755445066,1.40498873522851,0.20170989432247));
#10632=CARTESIAN_POINT('Ctrl Pts',(10.4952386855848,1.39414935393528,0.409096209702196));
#10633=CARTESIAN_POINT('Ctrl Pts',(10.4844020137689,1.3833101379008,0.616482542003833));
#10634=CARTESIAN_POINT('Ctrl Pts',(10.6031877991504,1.41093118264609,-0.00141083033817288));
#10635=CARTESIAN_POINT('Ctrl Pts',(10.5923442181457,1.40008262840665,0.205974657203891));
#10636=CARTESIAN_POINT('Ctrl Pts',(10.5815009048179,1.38923496752292,0.413360205434192));
#10637=CARTESIAN_POINT('Ctrl Pts',(10.5706576147941,1.37838663885266,0.62074571708141));
#10638=CARTESIAN_POINT('Ctrl Pts',(10.7489822201969,1.33286898269122,0.00215046584238339));
#10639=CARTESIAN_POINT('Ctrl Pts',(10.7381210493968,1.32201618867047,0.209534855263179));
#10640=CARTESIAN_POINT('Ctrl Pts',(10.7272598662103,1.31116338896628,0.416919242515175));
#10641=CARTESIAN_POINT('Ctrl Pts',(10.716398780155,1.30031077634578,0.624303643734563));
#10642=CARTESIAN_POINT('Ctrl Pts',(10.8001612475457,1.18151886169146,-0.00307678645922502));
#10643=CARTESIAN_POINT('Ctrl Pts',(10.7892926103682,1.17067663552019,0.20430785074418));
#10644=CARTESIAN_POINT('Ctrl Pts',(10.7784241800195,1.15983442267521,0.41169249890798));
#10645=CARTESIAN_POINT('Ctrl Pts',(10.7675555412906,1.14899250266155,0.619077151394146));
#10646=CARTESIAN_POINT('Ctrl Pts',(10.8003382383521,1.11671757294177,-0.00645397222975308));
#10647=CARTESIAN_POINT('Ctrl Pts',(10.7894696557425,1.1058798099729,0.200930938146656));
#10648=CARTESIAN_POINT('Ctrl Pts',(10.778601072647,1.09504222488243,0.408315857793383));
#10649=CARTESIAN_POINT('Ctrl Pts',(10.7677324890572,1.08420482079361,0.615700786872884));
#10650=CARTESIAN_POINT('Ctrl Pts',(10.5166159648474,1.4155315881283,3.37837396946483E-16));
#10651=CARTESIAN_POINT('Ctrl Pts',(10.5058777995597,1.40479094425298,0.205494164234944));
#10652=CARTESIAN_POINT('Ctrl Pts',(10.4951398148107,1.39405045994841,0.41098834481212));
#10653=CARTESIAN_POINT('Ctrl Pts',(10.4844020137689,1.3833101379008,0.616482542003833));
#10654=CARTESIAN_POINT('Ctrl Pts',(10.7677324890572,1.08420482079361,0.615700786872884));
#10655=CARTESIAN_POINT('Ctrl Pts',(10.7784883265195,1.09492980219801,0.410467182062988));
#10656=CARTESIAN_POINT('Ctrl Pts',(10.7892441634977,1.10565496086826,0.205233586491177));
#10657=CARTESIAN_POINT('Ctrl Pts',(10.8,1.11638029377732,-4.7271214720368E-17));
#10658=CARTESIAN_POINT('Ctrl Pts',(0.3318563713692,1.09142177001972,0.9));
#10659=CARTESIAN_POINT('Ctrl Pts',(1.77658538561441,1.20431139287985,0.9));
#10660=CARTESIAN_POINT('Ctrl Pts',(5.15852145577913,1.31798734362749,0.900000000000001));
#10661=CARTESIAN_POINT('Ctrl Pts',(8.53883158814675,1.18907590268945,0.9));
#10662=CARTESIAN_POINT('Ctrl Pts',(10.4681436286308,1.08420482079361,0.9));
#10663=CARTESIAN_POINT('Ctrl Pts',(0.325113511056836,1.17771496230318,0.9));
#10664=CARTESIAN_POINT('Ctrl Pts',(1.77238748853623,1.29094597754667,0.900005244311447));
#10665=CARTESIAN_POINT('Ctrl Pts',(5.15940689953628,1.40489117512763,0.899995532233175));
#10666=CARTESIAN_POINT('Ctrl Pts',(8.54259780483314,1.2757067056985,0.90000328531099));
#10667=CARTESIAN_POINT('Ctrl Pts',(10.4728449957889,1.17069581622255,0.9));
#10668=CARTESIAN_POINT('Ctrl Pts',(0.313425270489116,1.32729771265557,0.830156825336737));
#10669=CARTESIAN_POINT('Ctrl Pts',(1.76508272830699,1.44110107554431,0.829918234118879));
#10670=CARTESIAN_POINT('Ctrl Pts',(5.16095094050242,1.55552201031752,0.829677185710002));
#10671=CARTESIAN_POINT('Ctrl Pts',(8.54913632089268,1.4258591912674,0.829900861618366));
#10672=CARTESIAN_POINT('Ctrl Pts',(10.4809942371438,1.32061731204901,0.830050158657121));
#10673=CARTESIAN_POINT('Ctrl Pts',(0.308806004580394,1.38641375285276,0.681625057916928));
#10674=CARTESIAN_POINT('Ctrl Pts',(1.76222987578798,1.50017797416985,0.681006088930498));
#10675=CARTESIAN_POINT('Ctrl Pts',(5.16154986224672,1.61450132085358,0.68038246417749));
#10676=CARTESIAN_POINT('Ctrl Pts',(8.55170115551887,1.48491240850707,0.680961314820656));
#10677=CARTESIAN_POINT('Ctrl Pts',(10.4842082875648,1.37974615923803,0.681348425135383));
#10678=CARTESIAN_POINT('Ctrl Pts',(0.308522637995068,1.39004019713626,0.616809874278785));
#10679=CARTESIAN_POINT('Ctrl Pts',(1.76205965694675,1.50365920577193,0.616079089534579));
#10680=CARTESIAN_POINT('Ctrl Pts',(5.16158497046229,1.61783515152865,0.615338844765104));
#10681=CARTESIAN_POINT('Ctrl Pts',(8.55185322351876,1.48838233768137,0.616025627991778));
#10682=CARTESIAN_POINT('Ctrl Pts',(10.4844020137689,1.3833101379008,0.616482542003833));
#10683=CARTESIAN_POINT('Ctrl Pts',(10.4844020137689,1.3833101379008,0.616482542003833));
#10684=CARTESIAN_POINT('Ctrl Pts',(8.55185322351876,1.48838233768137,0.616025627991778));
#10685=CARTESIAN_POINT('Ctrl Pts',(5.16158497046229,1.61783515152865,0.615338844765104));
#10686=CARTESIAN_POINT('Ctrl Pts',(1.76205965694675,1.50365920577193,0.616079089534579));
#10687=CARTESIAN_POINT('Ctrl Pts',(0.308522637995068,1.39004019713626,0.616809874278785));
#10688=CARTESIAN_POINT('Ctrl Pts',(0.3318563713692,1.09142177001972,0.9));
#10689=CARTESIAN_POINT('Ctrl Pts',(1.77658538561441,1.20431139287985,0.9));
#10690=CARTESIAN_POINT('Ctrl Pts',(5.15852145577913,1.31798734362749,0.900000000000001));
#10691=CARTESIAN_POINT('Ctrl Pts',(8.53883158814675,1.18907590268945,0.9));
#10692=CARTESIAN_POINT('Ctrl Pts',(10.4681436286308,1.08420482079361,0.9));
#10693=CARTESIAN_POINT('Ctrl Pts',(-0.000344602063817145,1.12390349461883,
-0.00657539908256866));
#10694=CARTESIAN_POINT('Ctrl Pts',(0.0105261016091243,1.11307601020539,
0.200849983592616));
#10695=CARTESIAN_POINT('Ctrl Pts',(0.0213968059409475,1.10224876730309,
0.408275378840013));
#10696=CARTESIAN_POINT('Ctrl Pts',(0.0322675109428289,1.09142177001972,
0.615700786872884));
#10697=CARTESIAN_POINT('Ctrl Pts',(-0.000112549170678945,1.2089618047365,
-0.00214756610981592));
#10698=CARTESIAN_POINT('Ctrl Pts',(0.0107584275574203,1.19812589474889,
0.205277296000037));
#10699=CARTESIAN_POINT('Ctrl Pts',(0.021628504370896,1.18729063034778,0.412702239156743));
#10700=CARTESIAN_POINT('Ctrl Pts',(0.0324994852542487,1.17645511229507,
0.620127120417125));
#10701=CARTESIAN_POINT('Ctrl Pts',(0.0675181008536004,1.35659180908255,
0.00201426213057289));
#10702=CARTESIAN_POINT('Ctrl Pts',(0.0783748317004002,1.34574224493831,
0.20943904356877));
#10703=CARTESIAN_POINT('Ctrl Pts',(0.0892318011706237,1.33489254525337,
0.416863803530356));
#10704=CARTESIAN_POINT('Ctrl Pts',(0.100088380073201,1.32404321751407,0.624288602298589));
#10705=CARTESIAN_POINT('Ctrl Pts',(0.212439875011655,1.41741816253371,-0.00240566592686199));
#10706=CARTESIAN_POINT('Ctrl Pts',(0.223274062163905,1.40657840226088,0.20502076110302));
#10707=CARTESIAN_POINT('Ctrl Pts',(0.234108278795672,1.39573903465802,0.412447205628077));
#10708=CARTESIAN_POINT('Ctrl Pts',(0.244942059060342,1.38489960928785,0.619873667633733));
#10709=CARTESIAN_POINT('Ctrl Pts',(0.276041299849618,1.42253242682652,-0.00547191373834488));
#10710=CARTESIAN_POINT('Ctrl Pts',(0.286868655882245,1.41170146982041,0.201955326984501));
#10711=CARTESIAN_POINT('Ctrl Pts',(0.297695769965166,1.40087072543886,0.409382589539965));
#10712=CARTESIAN_POINT('Ctrl Pts',(0.308522637995069,1.39004019713626,0.616809874278785));
#10713=CARTESIAN_POINT('Ctrl Pts',(2.26869304592592E-17,1.12356026268968,
-3.16587034365767E-17));
#10714=CARTESIAN_POINT('Ctrl Pts',(0.0107558363321878,1.11284719399672,
0.205233583245308));
#10715=CARTESIAN_POINT('Ctrl Pts',(0.0215116733095221,1.10213436178043,
0.410467178800746));
#10716=CARTESIAN_POINT('Ctrl Pts',(0.0322675109428289,1.09142177001972,
0.615700786872884));
#10717=CARTESIAN_POINT('Ctrl Pts',(0.308522637995069,1.39004019713626,0.616809874278785));
#10718=CARTESIAN_POINT('Ctrl Pts',(0.297790973931072,1.40077548928706,0.411206561171438));
#10719=CARTESIAN_POINT('Ctrl Pts',(0.287059068122271,1.41151099373341,0.205603269859031));
#10720=CARTESIAN_POINT('Ctrl Pts',(0.276326924564681,1.42224670711126,-2.68882138776405E-16));
#10721=CARTESIAN_POINT('Ctrl Pts',(10.5166159648474,-1.4155315881283,0.));
#10722=CARTESIAN_POINT('Ctrl Pts',(10.5064062201588,-1.40475637621136,0.205603291426271));
#10723=CARTESIAN_POINT('Ctrl Pts',(10.4961964754701,-1.39398116429443,0.411206582852543));
#10724=CARTESIAN_POINT('Ctrl Pts',(10.4859867307814,-1.38320595237749,0.616809874278814));
#10725=CARTESIAN_POINT('Ctrl Pts',(7.10318628475318,-1.599994843061,0.));
#10726=CARTESIAN_POINT('Ctrl Pts',(7.09978773046573,-1.58921963114407,0.205603291426271));
#10727=CARTESIAN_POINT('Ctrl Pts',(7.09638917617828,-1.57844441922713,0.411206582852543));
#10728=CARTESIAN_POINT('Ctrl Pts',(7.09299062189083,-1.5676692073102,0.616809874278814));
#10729=CARTESIAN_POINT('Ctrl Pts',(3.68975660465893,-1.68747752195839,0.));
#10730=CARTESIAN_POINT('Ctrl Pts',(3.69316924077269,-1.67670231004145,0.205603291426272));
#10731=CARTESIAN_POINT('Ctrl Pts',(3.69658187688646,-1.66592709812452,0.411206582852543));
#10732=CARTESIAN_POINT('Ctrl Pts',(3.69999451300023,-1.65515188620758,0.616809874278814));
#10733=CARTESIAN_POINT('Ctrl Pts',(0.276326924564679,-1.42224670711126,
0.));
#10734=CARTESIAN_POINT('Ctrl Pts',(0.286550751079662,-1.41147149519433,
0.205603291426271));
#10735=CARTESIAN_POINT('Ctrl Pts',(0.296774577594646,-1.40069628327739,
0.411206582852543));
#10736=CARTESIAN_POINT('Ctrl Pts',(0.306998404109629,-1.38992107136046,
0.616809874278814));
#10737=CARTESIAN_POINT('Origin',(0.,-1.4,0.));
#10738=CARTESIAN_POINT('Origin',(5.4,-8.13935059369636E-18,0.9));
#10739=CARTESIAN_POINT('Ctrl Pts',(0.276326924564679,1.42224670711126,0.));
#10740=CARTESIAN_POINT('Ctrl Pts',(0.286550751079662,1.41147149519433,0.205603291426271));
#10741=CARTESIAN_POINT('Ctrl Pts',(0.296774577594645,1.40069628327739,0.411206582852543));
#10742=CARTESIAN_POINT('Ctrl Pts',(0.306998404109628,1.38992107136046,0.616809874278814));
#10743=CARTESIAN_POINT('Ctrl Pts',(3.68975660465893,1.68747752195839,0.));
#10744=CARTESIAN_POINT('Ctrl Pts',(3.6931692407727,1.67670231004145,0.205603291426271));
#10745=CARTESIAN_POINT('Ctrl Pts',(3.69658187688646,1.66592709812452,0.411206582852543));
#10746=CARTESIAN_POINT('Ctrl Pts',(3.69999451300023,1.65515188620758,0.616809874278814));
#10747=CARTESIAN_POINT('Ctrl Pts',(7.10318628475318,1.599994843061,0.));
#10748=CARTESIAN_POINT('Ctrl Pts',(7.09978773046573,1.58921963114407,0.205603291426271));
#10749=CARTESIAN_POINT('Ctrl Pts',(7.09638917617828,1.57844441922713,0.411206582852543));
#10750=CARTESIAN_POINT('Ctrl Pts',(7.09299062189083,1.5676692073102,0.616809874278814));
#10751=CARTESIAN_POINT('Ctrl Pts',(10.5166159648474,1.4155315881283,0.));
#10752=CARTESIAN_POINT('Ctrl Pts',(10.5064062201588,1.40475637621136,0.205603291426271));
#10753=CARTESIAN_POINT('Ctrl Pts',(10.4961964754701,1.39398116429443,0.411206582852543));
#10754=CARTESIAN_POINT('Ctrl Pts',(10.4859867307814,1.38320595237749,0.616809874278814));
#10755=CARTESIAN_POINT('Origin',(10.8,1.4,0.));
#18562=UNCERTAINTY_MEASURE_WITH_UNIT(LENGTH_MEASURE(0.001),#18581,
'DISTANCE_ACCURACY_VALUE',
'Maximum model space distance between geometric entities at asserted c
onnectivities');
#18568=UNCERTAINTY_MEASURE_WITH_UNIT(LENGTH_MEASURE(0.001),#18581,
'DISTANCE_ACCURACY_VALUE',
'Maximum model space distance between geometric entities at asserted c
onnectivities');
#18574=(
GEOMETRIC_REPRESENTATION_CONTEXT(3)
GLOBAL_UNCERTAINTY_ASSIGNED_CONTEXT((#18562))
GLOBAL_UNIT_ASSIGNED_CONTEXT((#18581,#18583,#18584))
REPRESENTATION_CONTEXT('','3D')
);
#18580=(
GEOMETRIC_REPRESENTATION_CONTEXT(3)
GLOBAL_UNCERTAINTY_ASSIGNED_CONTEXT((#18568))
GLOBAL_UNIT_ASSIGNED_CONTEXT((#18581,#18583,#18584))
REPRESENTATION_CONTEXT('','3D')
);
#18581=(
LENGTH_UNIT()
NAMED_UNIT(*)
SI_UNIT(.CENTI.,.METRE.)
);
#18583=(
NAMED_UNIT(*)
PLANE_ANGLE_UNIT()
SI_UNIT($,.RADIAN.)
);
#18584=(
NAMED_UNIT(*)
SI_UNIT($,.STERADIAN.)
SOLID_ANGLE_UNIT()
);
#18590=SHAPE_DEFINITION_REPRESENTATION(#18601,#18628);
#18601=PRODUCT_DEFINITION_SHAPE('',$,#18640);
#18628=SHAPE_REPRESENTATION('',(#6722),#18574);
#18634=PRODUCT_DEFINITION_CONTEXT('part definition',#18669,'design');
#18640=PRODUCT_DEFINITION('2026-11-10-05-09-36-725',
'Upper structural shell',#18651,#18634);
#18651=PRODUCT_DEFINITION_FORMATION('',$,#18676);
#18669=APPLICATION_CONTEXT(
'Core Data for Automotive Mechanical Design Process');
#18670=PRODUCT_CONTEXT('part definition',#18669,'mechanical');
#18676=PRODUCT('2026-11-10-05-09-36-725','Upper structural shell',$,(#18670));
#18686=PRESENTATION_STYLE_ASSIGNMENT((#18694));
#18694=SURFACE_STYLE_USAGE(.BOTH.,#18702);
#18702=SURFACE_SIDE_STYLE('',(#18710));
#18710=SURFACE_STYLE_FILL_AREA(#18718);
#18718=FILL_AREA_STYLE('Structural dark blue',(#18726));
#18726=FILL_AREA_STYLE_COLOUR('Structural dark blue',#18734);
#18734=COLOUR_RGB('Structural dark blue',0.0901960784313725,0.270588235294118,
0.513725490196078);
ENDSEC;
END-ISO-10303-21;
